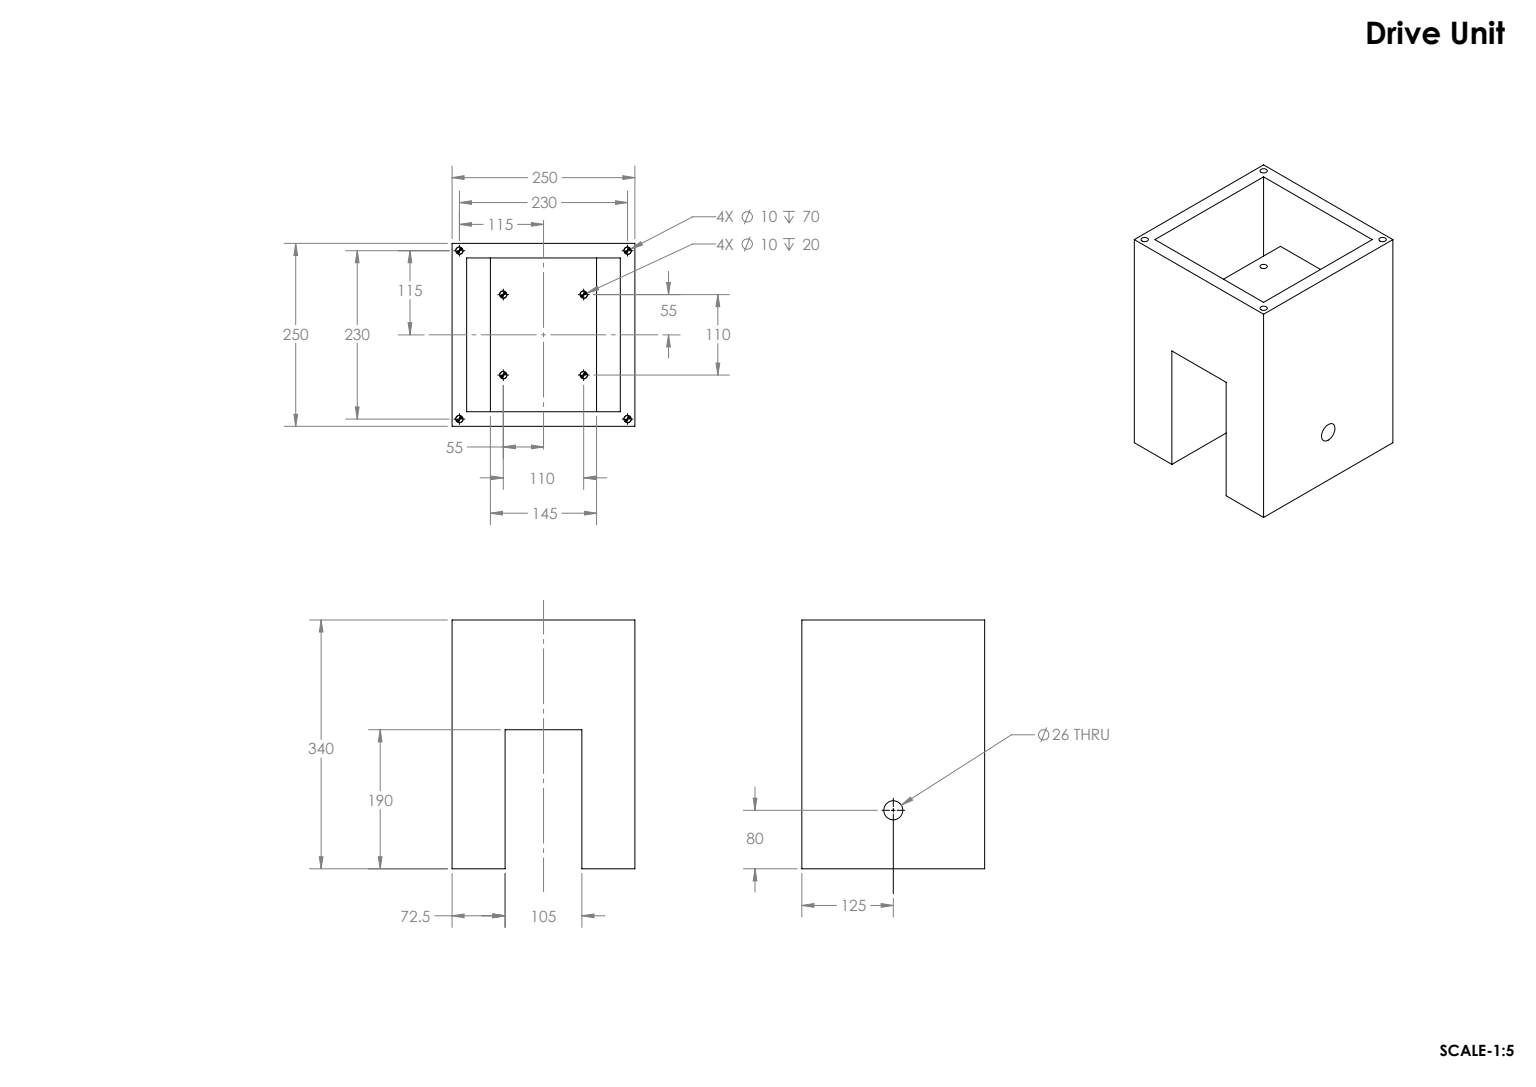
ISO-10303-21;
HEADER;
FILE_DESCRIPTION (('STEP AP214'),
    '1' );
FILE_NAME ('Drive Unit.step',
    '2026-10-28T15:55:38',
    ( '' ),
    ( '' ),
    'SwSTEP 2.0',
    'SolidWorks 2025',
    '' );
FILE_SCHEMA (( 'AUTOMOTIVE_DESIGN' ));
ENDSEC;

DATA;
#3=CARTESIAN_POINT ( 'NONE',  ( 125.0000000000000000, 52.50000000000000000, 190.0000000000000284 ) ) ;
#9=AXIS2_PLACEMENT_3D ( 'NONE', #2697, #3271, #106 ) ;
#13=ORIENTED_EDGE ( 'NONE', *, *, #6011, .T. ) ;
#17=CARTESIAN_POINT ( 'NONE',  ( 1.592040838891559490E-15, 125.0000000000000568, 92.99999999999992895 ) ) ;
#28=DIRECTION ( 'NONE',  ( -0.000000000000000000, -1.000000000000000000, 1.586032892321652236E-16 ) ) ;
#49=DIRECTION ( 'NONE',  ( -0.000000000000000000, -0.000000000000000000, 1.000000000000000000 ) ) ;
#55=ORIENTED_EDGE ( 'NONE', *, *, #309, .F. ) ;
#62=DIRECTION ( 'NONE',  ( -0.000000000000000000, -0.000000000000000000, 1.000000000000000000 ) ) ;
#63=FACE_OUTER_BOUND ( 'NONE', #5349, .T. ) ;
#67=VERTEX_POINT ( 'NONE', #6757 ) ;
#74=VECTOR ( 'NONE', #8127, 1000.000000000000000 ) ;
#78=LINE ( 'NONE', #2668, #2542 ) ;
#82=ORIENTED_EDGE ( 'NONE', *, *, #1098, .T. ) ;
#87=ADVANCED_FACE ( 'NONE', ( #1491 ), #7883, .F. ) ;
#93=DIRECTION ( 'NONE',  ( -0.000000000000000000, -1.460819769243626884E-16, -1.000000000000000000 ) ) ;
#94=SHAPE_REPRESENTATION_RELATIONSHIP ( 'NONE' , 'NONE' ,  #7203, #1812 ) ;
#98=VECTOR ( 'NONE', #4850, 1000.000000000000000 ) ;
#100=LINE ( 'NONE', #1995, #7998 ) ;
#102=DIRECTION ( 'NONE',  ( -0.000000000000000000, -0.000000000000000000, 1.000000000000000000 ) ) ;
#106=DIRECTION ( 'NONE',  ( 1.000000000000000000, 0.000000000000000000, 0.000000000000000000 ) ) ;
#109=CARTESIAN_POINT ( 'NONE',  ( -120.0000000000000000, 115.0000000000000000, 340.0000000000000000 ) ) ;
#112=VECTOR ( 'NONE', #2837, 1000.000000000000000 ) ;
#113=VECTOR ( 'NONE', #3248, 1000.000000000000000 ) ;
#120=CIRCLE ( 'NONE', #6870, 4.999999999999990230 ) ;
#123=FACE_OUTER_BOUND ( 'NONE', #4418, .T. ) ;
#124=ADVANCED_FACE ( 'NONE', ( #7222 ), #6594, .F. ) ;
#131=EDGE_CURVE ( 'NONE', #2948, #8274, #895, .T. ) ;
#136=CARTESIAN_POINT ( 'NONE',  ( -115.0000000000000142, 115.0000000000000000, 266.9956969048622568 ) ) ;
#137=ADVANCED_FACE ( 'NONE', ( #4082, #6676, #3444, #6029, #248 ), #2825, .F. ) ;
#145=DIRECTION ( 'NONE',  ( 1.000000000000000000, 0.000000000000000000, 0.000000000000000000 ) ) ;
#147=ORIENTED_EDGE ( 'NONE', *, *, #397, .F. ) ;
#149=DIRECTION ( 'NONE',  ( 0.000000000000000000, 0.000000000000000000, 1.000000000000000000 ) ) ;
#151=( NAMED_UNIT ( * ) PLANE_ANGLE_UNIT ( ) SI_UNIT ( $, .RADIAN. ) );
#152=EDGE_CURVE ( 'NONE', #6732, #6613, #6071, .T. ) ;
#157=ORIENTED_EDGE ( 'NONE', *, *, #4049, .T. ) ;
#162=DIRECTION ( 'NONE',  ( 0.000000000000000000, -1.224646799147353207E-16, 1.000000000000000000 ) ) ;
#164=DIRECTION ( 'NONE',  ( 0.000000000000000000, 1.224646799147353207E-16, -1.000000000000000000 ) ) ;
#168=CARTESIAN_POINT ( 'NONE',  ( -120.0000000000000000, 115.0000000000000000, 270.0000000000000000 ) ) ;
#171=CARTESIAN_POINT ( 'NONE',  ( 50.00000000000000711, 55.00000000000000000, 220.0000000000000284 ) ) ;
#174=CARTESIAN_POINT ( 'NONE',  ( -115.0000000000000000, 115.0000000000000000, 340.0000000000000000 ) ) ;
#184=LINE ( 'NONE', #4786, #3071 ) ;
#187=DIRECTION ( 'NONE',  ( -0.000000000000000000, -0.000000000000000000, 1.000000000000000000 ) ) ;
#193=ORIENTED_EDGE ( 'NONE', *, *, #2527, .T. ) ;
#199=DIRECTION ( 'NONE',  ( -0.000000000000000000, -1.632680918566406547E-16, -1.000000000000000000 ) ) ;
#205=( GEOMETRIC_REPRESENTATION_CONTEXT ( 3 ) GLOBAL_UNCERTAINTY_ASSIGNED_CONTEXT ( ( #320 ) ) GLOBAL_UNIT_ASSIGNED_CONTEXT ( ( #2718, #3942, #7322 ) ) REPRESENTATION_CONTEXT ( 'NONE', 'WORKASPACE' ) );
#214=DIRECTION ( 'NONE',  ( 1.000000000000000000, 0.000000000000000000, 0.000000000000000000 ) ) ;
#219=AXIS2_PLACEMENT_3D ( 'NONE', #1415, #5924, #6605 ) ;
#221=DIRECTION ( 'NONE',  ( -0.000000000000000000, -0.000000000000000000, 1.000000000000000000 ) ) ;
#223=ORIENTED_EDGE ( 'NONE', *, *, #4983, .T. ) ;
#224=CARTESIAN_POINT ( 'NONE',  ( 105.0000000000000000, 8.487013464091010249E-14, 20.00000000000001776 ) ) ;
#225=CARTESIAN_POINT ( 'NONE',  ( -125.0000000000000000, -125.0000000000000000, 340.0000000000000000 ) ) ;
#231=CONICAL_SURFACE ( 'NONE', #7932, 4.999999999999990230, 1.029744258676656754 ) ;
#233=PRODUCT_DEFINITION_CONTEXT ( 'detailed design', #2370, 'design' ) ;
#240=EDGE_CURVE ( 'NONE', #3849, #6134, #2101, .T. ) ;
#245=LINE ( 'NONE', #5564, #6769 ) ;
#247=CARTESIAN_POINT ( 'NONE',  ( 55.00000000000000000, 55.00000000000000000, 240.0000000000000284 ) ) ;
#248=FACE_OUTER_BOUND ( 'NONE', #5521, .T. ) ;
#255=CIRCLE ( 'NONE', #5116, 12.99999999999999822 ) ;
#256=DIRECTION ( 'NONE',  ( -1.000000000000000000, -1.321694076934710155E-16, 0.000000000000000000 ) ) ;
#260=VECTOR ( 'NONE', #1303, 1000.000000000000000 ) ;
#262=DIRECTION ( 'NONE',  ( -0.000000000000000000, -0.000000000000000000, 1.000000000000000000 ) ) ;
#264=EDGE_LOOP ( 'NONE', ( #6496, #2959, #7689, #1000 ) ) ;
#265=DIRECTION ( 'NONE',  ( 0.000000000000000000, 0.000000000000000000, -1.000000000000000000 ) ) ;
#266=LINE ( 'NONE', #3462, #5375 ) ;
#267=ORIENTED_EDGE ( 'NONE', *, *, #1486, .F. ) ;
#270=FACE_OUTER_BOUND ( 'NONE', #1601, .T. ) ;
#272=DIRECTION ( 'NONE',  ( 1.000000000000000000, 0.000000000000000000, 0.000000000000000000 ) ) ;
#276=CARTESIAN_POINT ( 'NONE',  ( -104.9999999999999432, -105.0000000000000853, 240.0000000000000284 ) ) ;
#279=CARTESIAN_POINT ( 'NONE',  ( 0.000000000000000000, 72.49999999999995737, 66.99999999999994316 ) ) ;
#287=CARTESIAN_POINT ( 'NONE',  ( 110.0000000000000142, -115.0000000000000000, 270.0000000000000000 ) ) ;
#289=CIRCLE ( 'NONE', #5015, 12.99999999999999822 ) ;
#292=ORIENTED_EDGE ( 'NONE', *, *, #3848, .F. ) ;
#297=PLANE ( 'NONE',  #642 ) ;
#303=CARTESIAN_POINT ( 'NONE',  ( 0.000000000000000000, 125.0000000000000568, 79.99999999999992895 ) ) ;
#309=EDGE_CURVE ( 'NONE', #7487, #6953, #643, .T. ) ;
#314=VERTEX_POINT ( 'NONE', #6672 ) ;
#320=UNCERTAINTY_MEASURE_WITH_UNIT (LENGTH_MEASURE( 1.000000000000000082E-05 ), #2718, 'distance_accuracy_value', 'NONE');
#323=VERTEX_POINT ( 'NONE', #4680 ) ;
#329=CARTESIAN_POINT ( 'NONE',  ( 120.0000000000000000, -115.0000000000000000, 270.0000000000000000 ) ) ;
#333=CARTESIAN_POINT ( 'NONE',  ( 125.0000000000000000, 52.50000000000000000, 190.0000000000000284 ) ) ;
#335=EDGE_CURVE ( 'NONE', #1946, #314, #6628, .T. ) ;
#336=ORIENTED_EDGE ( 'NONE', *, *, #3022, .F. ) ;
#344=CARTESIAN_POINT ( 'NONE',  ( 115.0000000000000000, 115.0000000000000000, 270.0000000000000000 ) ) ;
#345=DIRECTION ( 'NONE',  ( -0.000000000000000000, 1.000000000000000000, 1.224646799147353207E-16 ) ) ;
#346=EDGE_LOOP ( 'NONE', ( #3800, #3054, #6759, #1115 ) ) ;
#348=CARTESIAN_POINT ( 'NONE',  ( -115.0000000000000000, 115.0000000000000000, 340.0000000000000000 ) ) ;
#355=CARTESIAN_POINT ( 'NONE',  ( -110.0000000000000142, -115.0000000000000000, 270.0000000000000000 ) ) ;
#358=ORIENTED_EDGE ( 'NONE', *, *, #5305, .F. ) ;
#359=LINE ( 'NONE', #1094, #4691 ) ;
#360=ORIENTED_EDGE ( 'NONE', *, *, #2100, .T. ) ;
#366=DIRECTION ( 'NONE',  ( -0.000000000000000000, 1.000000000000000000, -0.000000000000000000 ) ) ;
#367=VECTOR ( 'NONE', #3652, 1000.000000000000000 ) ;
#368=ORIENTED_EDGE ( 'NONE', *, *, #2100, .F. ) ;
#373=CARTESIAN_POINT ( 'NONE',  ( 1.592040838891560279E-15, -125.0000000000000568, 92.99999999999997158 ) ) ;
#378=VERTEX_POINT ( 'NONE', #1356 ) ;
#385=EDGE_CURVE ( 'NONE', #378, #1211, #7861, .T. ) ;
#386=CARTESIAN_POINT ( 'NONE',  ( 105.0000000000000000, -105.0000000000000568, 240.0000000000000284 ) ) ;
#387=VECTOR ( 'NONE', #1755, 1000.000000000000000 ) ;
#397=EDGE_CURVE ( 'NONE', #2572, #1918, #4635, .T. ) ;
#416=VERTEX_POINT ( 'NONE', #5187 ) ;
#422=DIRECTION ( 'NONE',  ( -0.000000000000000000, -1.000000000000000000, -1.224646799147353207E-16 ) ) ;
#424=ORIENTED_EDGE ( 'NONE', *, *, #8219, .F. ) ;
#427=ORIENTED_EDGE ( 'NONE', *, *, #5038, .F. ) ;
#436=DIRECTION ( 'NONE',  ( -1.000000000000000000, -0.000000000000000000, -0.000000000000000000 ) ) ;
#439=DIRECTION ( 'NONE',  ( -0.000000000000000000, -0.000000000000000000, 1.000000000000000000 ) ) ;
#440=CARTESIAN_POINT ( 'NONE',  ( 1.592040838891560279E-15, -52.49999999999996447, 92.99999999999995737 ) ) ;
#443=EDGE_CURVE ( 'NONE', #5909, #448, #7758, .T. ) ;
#444=EDGE_CURVE ( 'NONE', #3837, #3210, #4518, .T. ) ;
#448=VERTEX_POINT ( 'NONE', #171 ) ;
#452=ORIENTED_EDGE ( 'NONE', *, *, #385, .T. ) ;
#454=ADVANCED_FACE ( 'NONE', ( #1334 ), #2234, .F. ) ;
#461=EDGE_CURVE ( 'NONE', #1211, #7416, #1823, .T. ) ;
#467=CARTESIAN_POINT ( 'NONE',  ( 0.000000000000000000, 72.49999999999995737, 79.99999999999994316 ) ) ;
#468=CYLINDRICAL_SURFACE ( 'NONE', #7813, 12.99999999999999822 ) ;
#469=VERTEX_POINT ( 'NONE', #7667 ) ;
#477=FACE_OUTER_BOUND ( 'NONE', #2938, .T. ) ;
#489=FACE_BOUND ( 'NONE', #5526, .T. ) ;
#503=DIRECTION ( 'NONE',  ( 1.000000000000000000, 1.321694076934710648E-16, 0.000000000000000000 ) ) ;
#508=ORIENTED_EDGE ( 'NONE', *, *, #4848, .F. ) ;
#509=VERTEX_POINT ( 'NONE', #329 ) ;
#510=EDGE_CURVE ( 'NONE', #4072, #3309, #2872, .T. ) ;
#513=DIRECTION ( 'NONE',  ( -0.000000000000000000, -0.000000000000000000, 1.000000000000000000 ) ) ;
#517=ORIENTED_EDGE ( 'NONE', *, *, #3189, .F. ) ;
#524=ORIENTED_EDGE ( 'NONE', *, *, #1693, .T. ) ;
#525=CIRCLE ( 'NONE', #6324, 4.999999999999990230 ) ;
#528=CARTESIAN_POINT ( 'NONE',  ( -55.00000000000000000, -55.00000000000000000, 220.0000000000000284 ) ) ;
#539=ORIENTED_EDGE ( 'NONE', *, *, #3641, .F. ) ;
#541=( GEOMETRIC_REPRESENTATION_CONTEXT ( 3 ) GLOBAL_UNCERTAINTY_ASSIGNED_CONTEXT ( ( #6320 ) ) GLOBAL_UNIT_ASSIGNED_CONTEXT ( ( #4638, #151, #7345 ) ) REPRESENTATION_CONTEXT ( 'NONE', 'WORKASPACE' ) );
#544=DIRECTION ( 'NONE',  ( -0.000000000000000000, -0.000000000000000000, 1.000000000000000000 ) ) ;
#549=VERTEX_POINT ( 'NONE', #6271 ) ;
#553=DIRECTION ( 'NONE',  ( -0.000000000000000000, -0.000000000000000000, 1.000000000000000000 ) ) ;
#556=CIRCLE ( 'NONE', #6891, 12.99999999999999822 ) ;
#564=CARTESIAN_POINT ( 'NONE',  ( -60.00000000000000000, 55.00000000000000000, 240.0000000000000284 ) ) ;
#568=DIRECTION ( 'NONE',  ( 1.000000000000000000, 0.000000000000000000, 0.000000000000000000 ) ) ;
#576=FACE_OUTER_BOUND ( 'NONE', #5063, .T. ) ;
#579=ADVANCED_FACE ( 'NONE', ( #2155 ), #2747, .F. ) ;
#580=ORIENTED_EDGE ( 'NONE', *, *, #3848, .T. ) ;
#591=ORIENTED_EDGE ( 'NONE', *, *, #4122, .F. ) ;
#603=LINE ( 'NONE', #4471, #650 ) ;
#605=DIRECTION ( 'NONE',  ( 1.000000000000000000, 0.000000000000000000, 0.000000000000000000 ) ) ;
#622=DIRECTION ( 'NONE',  ( -1.000000000000000000, 0.000000000000000000, -0.000000000000000000 ) ) ;
#623=ORIENTED_EDGE ( 'NONE', *, *, #2527, .F. ) ;
#624=VERTEX_POINT ( 'NONE', #5765 ) ;
#630=CARTESIAN_POINT ( 'NONE',  ( -105.0000000000000000, -72.49999999999994316, 20.00000000000002842 ) ) ;
#632=DIRECTION ( 'NONE',  ( 0.000000000000000000, -1.000000000000000000, 1.266875999117951024E-16 ) ) ;
#642=AXIS2_PLACEMENT_3D ( 'NONE', #2714, #6722, #256 ) ;
#643=LINE ( 'NONE', #4722, #6660 ) ;
#648=ORIENTED_EDGE ( 'NONE', *, *, #3135, .T. ) ;
#650=VECTOR ( 'NONE', #7306, 1000.000000000000000 ) ;
#651=ORIENTED_EDGE ( 'NONE', *, *, #7751, .F. ) ;
#657=PLANE ( 'NONE',  #5711 ) ;
#660=VECTOR ( 'NONE', #5010, 1000.000000000000000 ) ;
#679=VECTOR ( 'NONE', #7829, 1000.000000000000000 ) ;
#690=CARTESIAN_POINT ( 'NONE',  ( 0.000000000000000000, 72.49999999999995737, 79.99999999999994316 ) ) ;
#691=LINE ( 'NONE', #8174, #113 ) ;
#699=CARTESIAN_POINT ( 'NONE',  ( -55.00000000000000000, -55.00000000000000000, 220.0000000000000284 ) ) ;
#701=CARTESIAN_POINT ( 'NONE',  ( -60.00000000000000000, -55.00000000000000000, 240.0000000000000284 ) ) ;
#711=ORIENTED_EDGE ( 'NONE', *, *, #3187, .T. ) ;
#717=VERTEX_POINT ( 'NONE', #5434 ) ;
#726=CARTESIAN_POINT ( 'NONE',  ( 59.99999999999999289, 55.00000000000000000, 220.0000000000000284 ) ) ;
#728=DIRECTION ( 'NONE',  ( 0.000000000000000000, 0.000000000000000000, 1.000000000000000000 ) ) ;
#730=DIRECTION ( 'NONE',  ( -0.000000000000000000, 1.000000000000000000, 1.224646799147353207E-16 ) ) ;
#731=LINE ( 'NONE', #7181, #4203 ) ;
#736=CARTESIAN_POINT ( 'NONE',  ( 55.00000000000000000, 55.00000000000000000, 220.0000000000000284 ) ) ;
#746=FACE_OUTER_BOUND ( 'NONE', #7315, .T. ) ;
#747=EDGE_LOOP ( 'NONE', ( #539, #13, #8100 ) ) ;
#754=DIRECTION ( 'NONE',  ( 1.000000000000000000, 0.000000000000000000, 0.000000000000000000 ) ) ;
#762=DIRECTION ( 'NONE',  ( -1.000000000000000000, -0.000000000000000000, -0.000000000000000000 ) ) ;
#774=DIRECTION ( 'NONE',  ( 1.000000000000000000, 0.000000000000000000, 0.000000000000000000 ) ) ;
#782=DIRECTION ( 'NONE',  ( -0.000000000000000000, -0.000000000000000000, 1.000000000000000000 ) ) ;
#787=CIRCLE ( 'NONE', #5776, 4.999999999999997335 ) ;
#792=EDGE_CURVE ( 'NONE', #5384, #549, #5347, .T. ) ;
#798=FACE_BOUND ( 'NONE', #2089, .T. ) ;
#801=FACE_OUTER_BOUND ( 'NONE', #4380, .T. ) ;
#804=CARTESIAN_POINT ( 'NONE',  ( -115.0000000000000000, 115.0000000000000000, 340.0000000000000000 ) ) ;
#810=DIRECTION ( 'NONE',  ( 0.000000000000000000, -1.000000000000000000, -1.632680918566406547E-16 ) ) ;
#815=DIRECTION ( 'NONE',  ( -0.000000000000000000, -1.460819769243626884E-16, 1.000000000000000000 ) ) ;
#816=CIRCLE ( 'NONE', #7702, 4.999999999999990230 ) ;
#817=DIRECTION ( 'NONE',  ( 0.000000000000000000, 0.000000000000000000, -1.000000000000000000 ) ) ;
#821=DIRECTION ( 'NONE',  ( 1.000000000000000000, 0.000000000000000000, 0.000000000000000000 ) ) ;
#822=ORIENTED_EDGE ( 'NONE', *, *, #4122, .T. ) ;
#825=ORIENTED_EDGE ( 'NONE', *, *, #335, .F. ) ;
#839=LINE ( 'NONE', #6529, #4130 ) ;
#841=ORIENTED_EDGE ( 'NONE', *, *, #8140, .T. ) ;
#842=CIRCLE ( 'NONE', #983, 4.999999999999990230 ) ;
#851=CARTESIAN_POINT ( 'NONE',  ( 125.0000000000000000, -125.0000000000000000, 340.0000000000000000 ) ) ;
#852=DIRECTION ( 'NONE',  ( 1.000000000000000000, 0.000000000000000000, 0.000000000000000000 ) ) ;
#871=EDGE_CURVE ( 'NONE', #1109, #6237, #1148, .T. ) ;
#874=ADVANCED_FACE ( 'NONE', ( #1584 ), #2839, .F. ) ;
#876=DIRECTION ( 'NONE',  ( -0.000000000000000000, -1.460819769243626884E-16, 1.000000000000000000 ) ) ;
#879=CARTESIAN_POINT ( 'NONE',  ( 115.0000000000000000, 115.0000000000000000, 270.0000000000000000 ) ) ;
#884=ORIENTED_EDGE ( 'NONE', *, *, #4049, .F. ) ;
#889=CARTESIAN_POINT ( 'NONE',  ( 0.000000000000000000, -72.49999999999998579, 66.99999999999995737 ) ) ;
#890=PLANE ( 'NONE',  #4820 ) ;
#892=ADVANCED_FACE ( 'NONE', ( #5421 ), #4138, .F. ) ;
#895=LINE ( 'NONE', #5989, #5171 ) ;
#896=DIRECTION ( 'NONE',  ( 1.000000000000000000, 0.000000000000000000, 0.000000000000000000 ) ) ;
#903=FACE_OUTER_BOUND ( 'NONE', #8243, .T. ) ;
#907=VECTOR ( 'NONE', #3781, 1000.000000000000000 ) ;
#909=ORIENTED_EDGE ( 'NONE', *, *, #2279, .F. ) ;
#915=CARTESIAN_POINT ( 'NONE',  ( -105.0000000000000000, 8.487013464091010249E-14, 20.00000000000001776 ) ) ;
#922=EDGE_CURVE ( 'NONE', #6580, #3406, #3545, .T. ) ;
#923=VECTOR ( 'NONE', #513, 1000.000000000000000 ) ;
#942=DIRECTION ( 'NONE',  ( 0.000000000000000000, 0.000000000000000000, -1.000000000000000000 ) ) ;
#944=VECTOR ( 'NONE', #2401, 1000.000000000000000 ) ;
#952=VERTEX_POINT ( 'NONE', #3626 ) ;
#954=DIRECTION ( 'NONE',  ( 1.000000000000000000, 0.000000000000000000, 0.000000000000000000 ) ) ;
#962=EDGE_LOOP ( 'NONE', ( #5950, #591, #6803, #1518 ) ) ;
#963=ORIENTED_EDGE ( 'NONE', *, *, #1804, .T. ) ;
#972=ORIENTED_EDGE ( 'NONE', *, *, #2430, .F. ) ;
#977=DIRECTION ( 'NONE',  ( -0.000000000000000000, -0.000000000000000000, 1.000000000000000000 ) ) ;
#982=ADVANCED_FACE ( 'NONE', ( #4567 ), #7087, .F. ) ;
#983=AXIS2_PLACEMENT_3D ( 'NONE', #7682, #6478, #5268 ) ;
#1000=ORIENTED_EDGE ( 'NONE', *, *, #4569, .F. ) ;
#1001=DIRECTION ( 'NONE',  ( 1.000000000000000000, 0.000000000000000000, 0.000000000000000000 ) ) ;
#1008=VERTEX_POINT ( 'NONE', #7708 ) ;
#1017=DIRECTION ( 'NONE',  ( 0.000000000000000000, -1.224646799147353207E-16, 1.000000000000000000 ) ) ;
#1029=PLANE ( 'NONE',  #4537 ) ;
#1032=ORIENTED_EDGE ( 'NONE', *, *, #7372, .F. ) ;
#1033=AXIS2_PLACEMENT_3D ( 'NONE', #4475, #7026, #568 ) ;
#1034=ORIENTED_EDGE ( 'NONE', *, *, #3154, .F. ) ;
#1037=CARTESIAN_POINT ( 'NONE',  ( -115.0000000000000000, -115.0000000000000000, 340.0000000000000000 ) ) ;
#1038=ORIENTED_EDGE ( 'NONE', *, *, #5870, .T. ) ;
#1042=DIRECTION ( 'NONE',  ( 1.000000000000000000, 0.000000000000000000, 0.000000000000000000 ) ) ;
#1044=ORIENTED_EDGE ( 'NONE', *, *, #5451, .F. ) ;
#1050=CARTESIAN_POINT ( 'NONE',  ( -50.00000000000000000, -55.00000000000000000, 240.0000000000000284 ) ) ;
#1061=CARTESIAN_POINT ( 'NONE',  ( -105.0000000000000000, 8.487013464091010249E-14, 20.00000000000001776 ) ) ;
#1062=ORIENTED_EDGE ( 'NONE', *, *, #4848, .T. ) ;
#1067=EDGE_LOOP ( 'NONE', ( #3144, #1132, #360, #4244, #5256, #6664, #7467, #3226 ) ) ;
#1070=DIRECTION ( 'NONE',  ( 0.000000000000000000, 1.000000000000000000, -1.460819769243626884E-16 ) ) ;
#1082=AXIS2_PLACEMENT_3D ( 'NONE', #3202, #6495, #7747 ) ;
#1088=CARTESIAN_POINT ( 'NONE',  ( 0.000000000000000000, 125.0000000000000568, 79.99999999999992895 ) ) ;
#1093=VERTEX_POINT ( 'NONE', #4424 ) ;
#1094=CARTESIAN_POINT ( 'NONE',  ( 0.000000000000000000, 105.0000000000000568, 19.99999999999998934 ) ) ;
#1095=DIRECTION ( 'NONE',  ( 1.000000000000000000, 0.000000000000000000, 0.000000000000000000 ) ) ;
#1098=EDGE_CURVE ( 'NONE', #448, #3289, #5832, .T. ) ;
#1103=LINE ( 'NONE', #3662, #3498 ) ;
#1107=VECTOR ( 'NONE', #2087, 1000.000000000000000 ) ;
#1109=VERTEX_POINT ( 'NONE', #1317 ) ;
#1110=CARTESIAN_POINT ( 'NONE',  ( 110.0000000000000142, 115.0000000000000000, 270.0000000000000000 ) ) ;
#1112=VERTEX_POINT ( 'NONE', #1965 ) ;
#1115=ORIENTED_EDGE ( 'NONE', *, *, #3920, .T. ) ;
#1120=ORIENTED_EDGE ( 'NONE', *, *, #6894, .T. ) ;
#1122=DIRECTION ( 'NONE',  ( 0.000000000000000000, 0.000000000000000000, -1.000000000000000000 ) ) ;
#1123=VECTOR ( 'NONE', #1801, 1000.000000000000000 ) ;
#1132=ORIENTED_EDGE ( 'NONE', *, *, #5688, .T. ) ;
#1141=DIRECTION ( 'NONE',  ( 1.321694076934710648E-16, -1.000000000000000000, 0.000000000000000000 ) ) ;
#1148=CIRCLE ( 'NONE', #5858, 4.999999999999990230 ) ;
#1155=ORIENTED_EDGE ( 'NONE', *, *, #7137, .F. ) ;
#1166=LINE ( 'NONE', #2919, #1123 ) ;
#1168=DIRECTION ( 'NONE',  ( 1.000000000000000000, 0.000000000000000000, 0.000000000000000000 ) ) ;
#1195=ORIENTED_EDGE ( 'NONE', *, *, #7394, .T. ) ;
#1206=DIRECTION ( 'NONE',  ( -0.000000000000000000, -0.000000000000000000, 1.000000000000000000 ) ) ;
#1211=VERTEX_POINT ( 'NONE', #1443 ) ;
#1212=CARTESIAN_POINT ( 'NONE',  ( 1.592040838891560279E-15, 52.49999999999997868, 92.99999999999994316 ) ) ;
#1213=CIRCLE ( 'NONE', #4702, 12.99999999999999822 ) ;
#1218=CARTESIAN_POINT ( 'NONE',  ( 115.0000000000000000, -115.0000000000000000, 340.0000000000000000 ) ) ;
#1219=DIRECTION ( 'NONE',  ( 1.000000000000000000, 0.000000000000000000, 0.000000000000000000 ) ) ;
#1228=ORIENTED_EDGE ( 'NONE', *, *, #4164, .F. ) ;
#1231=PLANE ( 'NONE',  #1375 ) ;
#1232=ORIENTED_EDGE ( 'NONE', *, *, #6853, .T. ) ;
#1238=EDGE_LOOP ( 'NONE', ( #1678, #6258, #1261 ) ) ;
#1239=ORIENTED_EDGE ( 'NONE', *, *, #6373, .T. ) ;
#1243=EDGE_LOOP ( 'NONE', ( #8310, #7332 ) ) ;
#1244=AXIS2_PLACEMENT_3D ( 'NONE', #7131, #1351, #3234 ) ;
#1247=DIRECTION ( 'NONE',  ( 0.000000000000000000, 0.000000000000000000, 1.000000000000000000 ) ) ;
#1249=DIRECTION ( 'NONE',  ( 0.000000000000000000, -1.224646799147353207E-16, 1.000000000000000000 ) ) ;
#1250=ORIENTED_EDGE ( 'NONE', *, *, #444, .F. ) ;
#1251=DIRECTION ( 'NONE',  ( 0.000000000000000000, -1.000000000000000000, 1.586032892321652236E-16 ) ) ;
#1261=ORIENTED_EDGE ( 'NONE', *, *, #871, .T. ) ;
#1266=CARTESIAN_POINT ( 'NONE',  ( 110.0000000000000142, 115.0000000000000000, 270.0000000000000000 ) ) ;
#1279=DIRECTION ( 'NONE',  ( -1.000000000000000000, 0.000000000000000000, 0.000000000000000000 ) ) ;
#1283=EDGE_CURVE ( 'NONE', #5670, #323, #4893, .T. ) ;
#1289=DIRECTION ( 'NONE',  ( -0.000000000000000000, 1.266875999117951024E-16, 1.000000000000000000 ) ) ;
#1297=ORIENTED_EDGE ( 'NONE', *, *, #4699, .T. ) ;
#1299=AXIS2_PLACEMENT_3D ( 'NONE', #5884, #1507, #5927 ) ;
#1301=DIRECTION ( 'NONE',  ( 1.000000000000000000, 0.000000000000000000, 0.000000000000000000 ) ) ;
#1303=DIRECTION ( 'NONE',  ( -0.000000000000000000, -0.000000000000000000, 1.000000000000000000 ) ) ;
#1312=CARTESIAN_POINT ( 'NONE',  ( 0.000000000000000000, 125.0000000000000568, 79.99999999999992895 ) ) ;
#1317=CARTESIAN_POINT ( 'NONE',  ( 120.0000000000000000, 115.0000000000000000, 270.0000000000000000 ) ) ;
#1318=AXIS2_PLACEMENT_3D ( 'NONE', #2518, #49, #5807 ) ;
#1323=CARTESIAN_POINT ( 'NONE',  ( -55.00000000000000000, -55.00000000000000000, 240.0000000000000284 ) ) ;
#1324=CARTESIAN_POINT ( 'NONE',  ( 0.000000000000000000, 125.0000000000000568, 79.99999999999992895 ) ) ;
#1325=ORIENTED_EDGE ( 'NONE', *, *, #5972, .F. ) ;
#1326=FACE_OUTER_BOUND ( 'NONE', #4672, .T. ) ;
#1334=FACE_OUTER_BOUND ( 'NONE', #3551, .T. ) ;
#1337=CYLINDRICAL_SURFACE ( 'NONE', #2260, 12.99999999999999822 ) ;
#1342=ORIENTED_EDGE ( 'NONE', *, *, #2323, .F. ) ;
#1343=EDGE_CURVE ( 'NONE', #469, #717, #245, .T. ) ;
#1350=LINE ( 'NONE', #1266, #7264 ) ;
#1351=DIRECTION ( 'NONE',  ( -0.000000000000000000, -0.000000000000000000, 1.000000000000000000 ) ) ;
#1353=ORIENTED_EDGE ( 'NONE', *, *, #6378, .F. ) ;
#1355=ORIENTED_EDGE ( 'NONE', *, *, #1343, .T. ) ;
#1356=CARTESIAN_POINT ( 'NONE',  ( 54.99999999999999289, -55.00000000000000000, 216.9956969048622284 ) ) ;
#1357=EDGE_CURVE ( 'NONE', #3406, #6580, #842, .T. ) ;
#1369=CARTESIAN_POINT ( 'NONE',  ( 0.000000000000000000, 52.49999999999997868, 79.99999999999994316 ) ) ;
#1375=AXIS2_PLACEMENT_3D ( 'NONE', #6364, #3156, #632 ) ;
#1379=CARTESIAN_POINT ( 'NONE',  ( -59.99999999999999289, 55.00000000000000000, 220.0000000000000284 ) ) ;
#1383=ORIENTED_EDGE ( 'NONE', *, *, #1921, .F. ) ;
#1391=DIRECTION ( 'NONE',  ( -1.000000000000000000, -0.000000000000000000, 0.000000000000000000 ) ) ;
#1395=DIRECTION ( 'NONE',  ( -0.000000000000000000, -1.000000000000000000, -1.224646799147353207E-16 ) ) ;
#1415=CARTESIAN_POINT ( 'NONE',  ( 55.00000000000000000, -55.00000000000000000, 220.0000000000000284 ) ) ;
#1416=DIRECTION ( 'NONE',  ( 1.000000000000000000, 0.000000000000000000, 0.000000000000000000 ) ) ;
#1428=CYLINDRICAL_SURFACE ( 'NONE', #5906, 4.999999999999997335 ) ;
#1429=CARTESIAN_POINT ( 'NONE',  ( -55.00000000000000000, 55.00000000000000000, 240.0000000000000284 ) ) ;
#1443=CARTESIAN_POINT ( 'NONE',  ( 59.99999999999999289, -55.00000000000000000, 220.0000000000000284 ) ) ;
#1445=DIRECTION ( 'NONE',  ( -0.000000000000000000, -0.000000000000000000, 1.000000000000000000 ) ) ;
#1451=LINE ( 'NONE', #2709, #7830 ) ;
#1458=CARTESIAN_POINT ( 'NONE',  ( 125.0000000000000000, 52.49999999999997158, 0.000000000000000000 ) ) ;
#1459=DIRECTION ( 'NONE',  ( -0.000000000000000000, -0.000000000000000000, 1.000000000000000000 ) ) ;
#1469=CARTESIAN_POINT ( 'NONE',  ( -55.00000000000000000, -55.00000000000000000, 220.0000000000000284 ) ) ;
#1475=AXIS2_PLACEMENT_3D ( 'NONE', #1369, #3932, #5873 ) ;
#1480=AXIS2_PLACEMENT_3D ( 'NONE', #386, #2871, #1541 ) ;
#1486=EDGE_CURVE ( 'NONE', #3309, #4072, #289, .T. ) ;
#1489=CARTESIAN_POINT ( 'NONE',  ( -125.0000000000000000, -52.50000000000000000, 190.0000000000000284 ) ) ;
#1491=FACE_OUTER_BOUND ( 'NONE', #747, .T. ) ;
#1496=EDGE_LOOP ( 'NONE', ( #3327, #3854, #5221 ) ) ;
#1507=DIRECTION ( 'NONE',  ( 0.000000000000000000, 0.000000000000000000, 1.000000000000000000 ) ) ;
#1512=CIRCLE ( 'NONE', #6214, 4.999999999999990230 ) ;
#1518=ORIENTED_EDGE ( 'NONE', *, *, #5972, .T. ) ;
#1520=ORIENTED_EDGE ( 'NONE', *, *, #3187, .F. ) ;
#1534=VERTEX_POINT ( 'NONE', #2242 ) ;
#1536=AXIS2_PLACEMENT_3D ( 'NONE', #4125, #942, #3490 ) ;
#1539=DIRECTION ( 'NONE',  ( 1.000000000000000000, 0.000000000000000000, 0.000000000000000000 ) ) ;
#1541=DIRECTION ( 'NONE',  ( 0.000000000000000000, 0.000000000000000000, -1.000000000000000000 ) ) ;
#1544=LINE ( 'NONE', #6081, #387 ) ;
#1547=LINE ( 'NONE', #2193, #3061 ) ;
#1551=FACE_OUTER_BOUND ( 'NONE', #7596, .T. ) ;
#1553=ORIENTED_EDGE ( 'NONE', *, *, #1693, .F. ) ;
#1556=EDGE_CURVE ( 'NONE', #1093, #3982, #1166, .T. ) ;
#1562=VERTEX_POINT ( 'NONE', #8172 ) ;
#1571=DIRECTION ( 'NONE',  ( 0.000000000000000000, -1.224646799147353207E-16, 1.000000000000000000 ) ) ;
#1575=DIRECTION ( 'NONE',  ( -0.000000000000000000, 1.266875999117951024E-16, 1.000000000000000000 ) ) ;
#1584=FACE_OUTER_BOUND ( 'NONE', #7774, .T. ) ;
#1588=ORIENTED_EDGE ( 'NONE', *, *, #3237, .T. ) ;
#1591=AXIS2_PLACEMENT_3D ( 'NONE', #3931, #5710, #6978 ) ;
#1596=CARTESIAN_POINT ( 'NONE',  ( -55.00000000000000000, -55.00000000000000000, 220.0000000000000284 ) ) ;
#1597=AXIS2_PLACEMENT_3D ( 'NONE', #4723, #1445, #2133 ) ;
#1601=EDGE_LOOP ( 'NONE', ( #2907, #8094, #822 ) ) ;
#1604=AXIS2_PLACEMENT_3D ( 'NONE', #4532, #7083, #1301 ) ;
#1622=AXIS2_PLACEMENT_3D ( 'NONE', #2587, #6337, #5791 ) ;
#1628=DIRECTION ( 'NONE',  ( 0.000000000000000000, 0.000000000000000000, -1.000000000000000000 ) ) ;
#1629=FACE_OUTER_BOUND ( 'NONE', #264, .T. ) ;
#1630=ORIENTED_EDGE ( 'NONE', *, *, #7051, .T. ) ;
#1637=ORIENTED_EDGE ( 'NONE', *, *, #444, .T. ) ;
#1643=EDGE_CURVE ( 'NONE', #6249, #5775, #7359, .T. ) ;
#1647=EDGE_CURVE ( 'NONE', #4789, #3289, #5301, .T. ) ;
#1648=ORIENTED_EDGE ( 'NONE', *, *, #5870, .F. ) ;
#1649=DIRECTION ( 'NONE',  ( 0.8571673007021134438, 0.000000000000000000, 0.5150380749100522682 ) ) ;
#1658=FACE_OUTER_BOUND ( 'NONE', #1067, .T. ) ;
#1665=VERTEX_POINT ( 'NONE', #7350 ) ;
#1671=EDGE_LOOP ( 'NONE', ( #3004, #2889, #8068, #4799 ) ) ;
#1672=CYLINDRICAL_SURFACE ( 'NONE', #4564, 12.99999999999999822 ) ;
#1676=DIRECTION ( 'NONE',  ( 1.000000000000000000, 0.000000000000000000, 0.000000000000000000 ) ) ;
#1678=ORIENTED_EDGE ( 'NONE', *, *, #6853, .F. ) ;
#1690=CARTESIAN_POINT ( 'NONE',  ( -115.0000000000000000, -115.0000000000000000, 270.0000000000000000 ) ) ;
#1693=EDGE_CURVE ( 'NONE', #5775, #2457, #5565, .T. ) ;
#1709=AXIS2_PLACEMENT_3D ( 'NONE', #4046, #7188, #5252 ) ;
#1710=ORIENTED_EDGE ( 'NONE', *, *, #6741, .T. ) ;
#1716=CARTESIAN_POINT ( 'NONE',  ( -115.0000000000000000, 115.0000000000000000, 270.0000000000000000 ) ) ;
#1722=ORIENTED_EDGE ( 'NONE', *, *, #7897, .T. ) ;
#1723=LINE ( 'NONE', #4756, #3086 ) ;
#1726=CARTESIAN_POINT ( 'NONE',  ( 125.0000000000000000, 125.0000000000000568, -9.184850993605156622E-15 ) ) ;
#1736=VECTOR ( 'NONE', #7864, 1000.000000000000000 ) ;
#1737=ORIENTED_EDGE ( 'NONE', *, *, #443, .F. ) ;
#1753=LINE ( 'NONE', #2434, #2301 ) ;
#1755=DIRECTION ( 'NONE',  ( -1.000000000000000000, 0.000000000000000000, 0.000000000000000000 ) ) ;
#1757=ADVANCED_FACE ( 'NONE', ( #3722 ), #3166, .F. ) ;
#1759=EDGE_CURVE ( 'NONE', #3837, #1946, #3323, .T. ) ;
#1775=CARTESIAN_POINT ( 'NONE',  ( 0.000000000000000000, -125.0000000000000568, 79.99999999999997158 ) ) ;
#1782=ORIENTED_EDGE ( 'NONE', *, *, #6074, .T. ) ;
#1786=AXIS2_PLACEMENT_3D ( 'NONE', #8007, #8046, #272 ) ;
#1796=CARTESIAN_POINT ( 'NONE',  ( 105.0000000000000000, -105.0000000000000568, 240.0000000000000284 ) ) ;
#1801=DIRECTION ( 'NONE',  ( 1.000000000000000000, 0.000000000000000000, 0.000000000000000000 ) ) ;
#1804=EDGE_CURVE ( 'NONE', #378, #7416, #731, .T. ) ;
#1806=EDGE_CURVE ( 'NONE', #4162, #3924, #4896, .T. ) ;
#1809=VECTOR ( 'NONE', #3841, 1000.000000000000000 ) ;
#1810=ORIENTED_EDGE ( 'NONE', *, *, #5085, .T. ) ;
#1812=ADVANCED_BREP_SHAPE_REPRESENTATION ( '', ( #6502, #1299 ), #205 ) ;
#1816=ORIENTED_EDGE ( 'NONE', *, *, #1283, .T. ) ;
#1819=CARTESIAN_POINT ( 'NONE',  ( 120.0000000000000000, -115.0000000000000000, 340.0000000000000000 ) ) ;
#1823=CIRCLE ( 'NONE', #3960, 4.999999999999990230 ) ;
#1837=ORIENTED_EDGE ( 'NONE', *, *, #3482, .T. ) ;
#1839=FACE_OUTER_BOUND ( 'NONE', #7122, .T. ) ;
#1840=DIRECTION ( 'NONE',  ( -0.000000000000000000, -1.000000000000000000, 1.586032892321652236E-16 ) ) ;
#1847=DIRECTION ( 'NONE',  ( -0.000000000000000000, -1.000000000000000000, 1.586032892321652236E-16 ) ) ;
#1857=DIRECTION ( 'NONE',  ( -0.8571673007021116675, 1.049727191138617833E-16, 0.5150380749100552658 ) ) ;
#1862=ORIENTED_EDGE ( 'NONE', *, *, #6074, .F. ) ;
#1872=CARTESIAN_POINT ( 'NONE',  ( 120.0000000000000000, -115.0000000000000000, 340.0000000000000000 ) ) ;
#1875=LINE ( 'NONE', #5150, #6737 ) ;
#1877=AXIS2_PLACEMENT_3D ( 'NONE', #1596, #5896, #7892 ) ;
#1878=VERTEX_POINT ( 'NONE', #6800 ) ;
#1893=CIRCLE ( 'NONE', #2163, 4.999999999999990230 ) ;
#1904=VERTEX_POINT ( 'NONE', #7572 ) ;
#1911=ORIENTED_EDGE ( 'NONE', *, *, #7216, .T. ) ;
#1918=VERTEX_POINT ( 'NONE', #7219 ) ;
#1921=EDGE_CURVE ( 'NONE', #67, #5909, #2099, .T. ) ;
#1922=ADVANCED_FACE ( 'NONE', ( #2703, #5284 ), #890, .F. ) ;
#1929=DIRECTION ( 'NONE',  ( -0.000000000000000000, 0.000000000000000000, 1.000000000000000000 ) ) ;
#1935=VERTEX_POINT ( 'NONE', #5949 ) ;
#1946=VERTEX_POINT ( 'NONE', #4719 ) ;
#1950=CARTESIAN_POINT ( 'NONE',  ( -50.00000000000000711, -55.00000000000000000, 220.0000000000000284 ) ) ;
#1951=EDGE_LOOP ( 'NONE', ( #3758, #5816, #825, #2312 ) ) ;
#1953=CARTESIAN_POINT ( 'NONE',  ( 1.592040838891559490E-15, 125.0000000000000568, 92.99999999999992895 ) ) ;
#1954=CARTESIAN_POINT ( 'NONE',  ( -104.9999999999999432, -105.0000000000000853, 240.0000000000000284 ) ) ;
#1960=CARTESIAN_POINT ( 'NONE',  ( 59.99999999999999289, -55.00000000000000000, 220.0000000000000284 ) ) ;
#1961=CYLINDRICAL_SURFACE ( 'NONE', #4815, 4.999999999999990230 ) ;
#1964=DIRECTION ( 'NONE',  ( 1.000000000000000000, 0.000000000000000000, 0.000000000000000000 ) ) ;
#1965=CARTESIAN_POINT ( 'NONE',  ( -120.0000000000000000, 115.0000000000000000, 270.0000000000000000 ) ) ;
#1972=CARTESIAN_POINT ( 'NONE',  ( 0.000000000000000000, -72.49999999999994316, -212.5000000000000568 ) ) ;
#1974=ORIENTED_EDGE ( 'NONE', *, *, #2868, .T. ) ;
#1995=CARTESIAN_POINT ( 'NONE',  ( 125.0000000000000000, -52.50000000000000000, 190.0000000000000284 ) ) ;
#1997=ORIENTED_EDGE ( 'NONE', *, *, #2026, .T. ) ;
#2004=CARTESIAN_POINT ( 'NONE',  ( 55.00000000000000000, 55.00000000000000000, 220.0000000000000284 ) ) ;
#2006=ORIENTED_EDGE ( 'NONE', *, *, #8312, .F. ) ;
#2012=CARTESIAN_POINT ( 'NONE',  ( 105.0000000000000000, 72.49999999999994316, 240.0000000000000284 ) ) ;
#2014=CIRCLE ( 'NONE', #6979, 12.99999999999999822 ) ;
#2020=DIRECTION ( 'NONE',  ( -0.8571673007021134438, 1.049727191138620051E-16, 0.5150380749100522682 ) ) ;
#2026=EDGE_CURVE ( 'NONE', #6580, #5343, #5986, .T. ) ;
#2031=AXIS2_PLACEMENT_3D ( 'NONE', #2189, #4740, #7321 ) ;
#2032=EDGE_CURVE ( 'NONE', #6276, #1109, #7478, .T. ) ;
#2035=CARTESIAN_POINT ( 'NONE',  ( -105.0000000000000000, 72.49999999999994316, 240.0000000000000284 ) ) ;
#2049=CARTESIAN_POINT ( 'NONE',  ( 55.00000000000000000, -55.00000000000000000, 240.0000000000000284 ) ) ;
#2051=EDGE_LOOP ( 'NONE', ( #4977, #6871 ) ) ;
#2057=ORIENTED_EDGE ( 'NONE', *, *, #4536, .F. ) ;
#2067=CARTESIAN_POINT ( 'NONE',  ( -120.0000000000000000, -115.0000000000000000, 340.0000000000000000 ) ) ;
#2072=CARTESIAN_POINT ( 'NONE',  ( -125.0000000000000000, 52.50000000000000000, 190.0000000000000284 ) ) ;
#2074=CARTESIAN_POINT ( 'NONE',  ( 125.0000000000000000, -52.49999999999997158, 0.000000000000000000 ) ) ;
#2081=EDGE_LOOP ( 'NONE', ( #147, #6748, #1034, #3870, #55, #6533, #2869, #3571 ) ) ;
#2087=DIRECTION ( 'NONE',  ( 0.8571673007021134438, 0.000000000000000000, 0.5150380749100522682 ) ) ;
#2088=EDGE_CURVE ( 'NONE', #2457, #5057, #5401, .T. ) ;
#2089=EDGE_LOOP ( 'NONE', ( #2586, #7609 ) ) ;
#2099=LINE ( 'NONE', #726, #1736 ) ;
#2100=EDGE_CURVE ( 'NONE', #469, #8240, #4120, .T. ) ;
#2101=CIRCLE ( 'NONE', #4632, 12.99999999999999822 ) ;
#2105=EDGE_CURVE ( 'NONE', #5395, #2109, #556, .T. ) ;
#2106=CARTESIAN_POINT ( 'NONE',  ( -55.00000000000000000, 55.00000000000000000, 240.0000000000000284 ) ) ;
#2109=VERTEX_POINT ( 'NONE', #2259 ) ;
#2113=CARTESIAN_POINT ( 'NONE',  ( -104.9999999999999432, -105.0000000000000853, 240.0000000000000284 ) ) ;
#2124=AXIS2_PLACEMENT_3D ( 'NONE', #6427, #3220, #2606 ) ;
#2127=CIRCLE ( 'NONE', #6821, 4.999999999999997335 ) ;
#2131=VECTOR ( 'NONE', #8255, 1000.000000000000000 ) ;
#2133=DIRECTION ( 'NONE',  ( 1.000000000000000000, 0.000000000000000000, 0.000000000000000000 ) ) ;
#2144=VECTOR ( 'NONE', #28, 1000.000000000000000 ) ;
#2155=FACE_OUTER_BOUND ( 'NONE', #1496, .T. ) ;
#2156=ORIENTED_EDGE ( 'NONE', *, *, #4836, .T. ) ;
#2158=DIRECTION ( 'NONE',  ( -0.000000000000000000, -0.000000000000000000, 1.000000000000000000 ) ) ;
#2160=VECTOR ( 'NONE', #1857, 1000.000000000000000 ) ;
#2163=AXIS2_PLACEMENT_3D ( 'NONE', #528, #8221, #1168 ) ;
#2164=EDGE_CURVE ( 'NONE', #6732, #509, #7739, .T. ) ;
#2167=ORIENTED_EDGE ( 'NONE', *, *, #4580, .T. ) ;
#2171=ADVANCED_FACE ( 'NONE', ( #4410 ), #1231, .T. ) ;
#2172=EDGE_CURVE ( 'NONE', #1878, #7656, #1103, .T. ) ;
#2173=CARTESIAN_POINT ( 'NONE',  ( 60.00000000000000000, 55.00000000000000000, 240.0000000000000284 ) ) ;
#2175=AXIS2_PLACEMENT_3D ( 'NONE', #1726, #1575, #3608 ) ;
#2176=DIRECTION ( 'NONE',  ( 0.000000000000000000, 0.000000000000000000, -1.000000000000000000 ) ) ;
#2177=CARTESIAN_POINT ( 'NONE',  ( -115.0000000000000000, 115.0000000000000000, 270.0000000000000000 ) ) ;
#2182=ORIENTED_EDGE ( 'NONE', *, *, #3572, .F. ) ;
#2189=CARTESIAN_POINT ( 'NONE',  ( -115.0000000000000000, 115.0000000000000000, 270.0000000000000000 ) ) ;
#2190=VECTOR ( 'NONE', #366, 1000.000000000000000 ) ;
#2193=CARTESIAN_POINT ( 'NONE',  ( 105.0000000000000000, -105.0000000000000568, 240.0000000000000284 ) ) ;
#2199=EDGE_LOOP ( 'NONE', ( #7443, #8010, #5457 ) ) ;
#2203=DIRECTION ( 'NONE',  ( 0.000000000000000000, -1.000000000000000000, -1.460819769243626884E-16 ) ) ;
#2206=EDGE_LOOP ( 'NONE', ( #2331, #1250, #6833, #157 ) ) ;
#2230=CLOSED_SHELL ( 'NONE', ( #7292, #3818, #3695, #7103, #892, #4170, #7703, #2485, #7938, #579, #5920, #3689, #2276, #4404, #6905, #7013, #3012, #1757, #8269, #874, #137, #7115, #5151, #2721, #6602, #124, #3198, #4584, #3574, #8030, #1922, #2630, #6400, #4513, #2249, #7480, #6634, #7438, #4322, #3235, #7023, #2366, #4996, #982, #4732, #3586, #2579, #6350, #4357, #454, #5774, #3175, #5137, #87, #5192, #7718, #2171, #2926, #7211 ) ) ;
#2234=CONICAL_SURFACE ( 'NONE', #7068, 4.999999999999990230, 1.029744258676656754 ) ;
#2242=CARTESIAN_POINT ( 'NONE',  ( 110.0000000000000142, -115.0000000000000000, 340.0000000000000000 ) ) ;
#2244=ORIENTED_EDGE ( 'NONE', *, *, #7704, .F. ) ;
#2245=DIRECTION ( 'NONE',  ( 1.000000000000000000, 0.000000000000000000, 0.000000000000000000 ) ) ;
#2248=FACE_OUTER_BOUND ( 'NONE', #5783, .T. ) ;
#2249=ADVANCED_FACE ( 'NONE', ( #7931 ), #5823, .T. ) ;
#2251=CARTESIAN_POINT ( 'NONE',  ( 115.0000000000000000, -115.0000000000000000, 270.0000000000000000 ) ) ;
#2254=DIRECTION ( 'NONE',  ( -1.000000000000000000, 0.000000000000000000, 0.000000000000000000 ) ) ;
#2259=CARTESIAN_POINT ( 'NONE',  ( 1.592040838891560279E-15, 105.0000000000000426, 92.99999999999992895 ) ) ;
#2260=AXIS2_PLACEMENT_3D ( 'NONE', #3141, #1847, #7677 ) ;
#2268=EDGE_CURVE ( 'NONE', #1008, #7487, #3989, .T. ) ;
#2276=ADVANCED_FACE ( 'NONE', ( #2658 ), #2766, .F. ) ;
#2279=EDGE_CURVE ( 'NONE', #8276, #5343, #7442, .T. ) ;
#2280=DIRECTION ( 'NONE',  ( -0.000000000000000000, -0.000000000000000000, 1.000000000000000000 ) ) ;
#2281=ORIENTED_EDGE ( 'NONE', *, *, #4563, .F. ) ;
#2284=CARTESIAN_POINT ( 'NONE',  ( 105.0000000000000000, 105.0000000000000568, 240.0000000000000284 ) ) ;
#2285=CARTESIAN_POINT ( 'NONE',  ( 115.0000000000000000, -115.0000000000000000, 270.0000000000000000 ) ) ;
#2290=VECTOR ( 'NONE', #3868, 1000.000000000000000 ) ;
#2297=AXIS2_PLACEMENT_3D ( 'NONE', #1037, #7497, #6690 ) ;
#2299=LINE ( 'NONE', #1061, #98 ) ;
#2301=VECTOR ( 'NONE', #7577, 1000.000000000000000 ) ;
#2305=ORIENTED_EDGE ( 'NONE', *, *, #3755, .F. ) ;
#2312=ORIENTED_EDGE ( 'NONE', *, *, #5305, .T. ) ;
#2319=EDGE_LOOP ( 'NONE', ( #6583, #1120, #8295, #4661 ) ) ;
#2321=LINE ( 'NONE', #2931, #7030 ) ;
#2322=EDGE_CURVE ( 'NONE', #3289, #4789, #5282, .T. ) ;
#2323=EDGE_CURVE ( 'NONE', #6249, #2457, #3389, .T. ) ;
#2326=EDGE_LOOP ( 'NONE', ( #4674, #6501, #5921, #1911 ) ) ;
#2331=ORIENTED_EDGE ( 'NONE', *, *, #2487, .T. ) ;
#2334=DIRECTION ( 'NONE',  ( 0.000000000000000000, 0.000000000000000000, -1.000000000000000000 ) ) ;
#2339=ORIENTED_EDGE ( 'NONE', *, *, #7540, .T. ) ;
#2347=CARTESIAN_POINT ( 'NONE',  ( 125.0000000000000000, 0.000000000000000000, 0.000000000000000000 ) ) ;
#2349=LINE ( 'NONE', #6211, #112 ) ;
#2359=DIRECTION ( 'NONE',  ( -0.000000000000000000, -0.000000000000000000, 1.000000000000000000 ) ) ;
#2365=ORIENTED_EDGE ( 'NONE', *, *, #2427, .F. ) ;
#2366=ADVANCED_FACE ( 'NONE', ( #801 ), #8108, .F. ) ;
#2370=APPLICATION_CONTEXT ( 'automotive_design' ) ;
#2376=EDGE_LOOP ( 'NONE', ( #6968, #5734 ) ) ;
#2393=AXIS2_PLACEMENT_3D ( 'NONE', #3814, #2436, #6465 ) ;
#2397=DIRECTION ( 'NONE',  ( -0.000000000000000000, -0.000000000000000000, 1.000000000000000000 ) ) ;
#2401=DIRECTION ( 'NONE',  ( 0.000000000000000000, -1.000000000000000000, 1.266875999117951024E-16 ) ) ;
#2407=AXIS2_PLACEMENT_3D ( 'NONE', #3647, #6226, #1219 ) ;
#2411=ORIENTED_EDGE ( 'NONE', *, *, #2860, .F. ) ;
#2416=VECTOR ( 'NONE', #4711, 1000.000000000000000 ) ;
#2419=ORIENTED_EDGE ( 'NONE', *, *, #3638, .T. ) ;
#2427=EDGE_CURVE ( 'NONE', #1534, #3826, #1512, .T. ) ;
#2430=EDGE_CURVE ( 'NONE', #509, #6613, #6898, .T. ) ;
#2432=AXIS2_PLACEMENT_3D ( 'NONE', #1469, #102, #7333 ) ;
#2434=CARTESIAN_POINT ( 'NONE',  ( 0.000000000000000000, 125.0000000000000568, 66.99999999999992895 ) ) ;
#2436=DIRECTION ( 'NONE',  ( -0.000000000000000000, -0.000000000000000000, 1.000000000000000000 ) ) ;
#2438=AXIS2_PLACEMENT_3D ( 'NONE', #7024, #1206, #605 ) ;
#2448=ORIENTED_EDGE ( 'NONE', *, *, #3237, .F. ) ;
#2457=VERTEX_POINT ( 'NONE', #355 ) ;
#2458=CARTESIAN_POINT ( 'NONE',  ( -59.99999999999999289, -55.00000000000000000, 220.0000000000000284 ) ) ;
#2461=ORIENTED_EDGE ( 'NONE', *, *, #7161, .F. ) ;
#2468=EDGE_LOOP ( 'NONE', ( #1239, #4779, #1155, #3877, #4051, #5086, #6552, #1588 ) ) ;
#2476=DIRECTION ( 'NONE',  ( 0.000000000000000000, 1.460819769243626884E-16, 1.000000000000000000 ) ) ;
#2485=ADVANCED_FACE ( 'NONE', ( #6057 ), #4862, .F. ) ;
#2487=EDGE_CURVE ( 'NONE', #6953, #3210, #2321, .T. ) ;
#2492=EDGE_LOOP ( 'NONE', ( #7433, #292 ) ) ;
#2493=CARTESIAN_POINT ( 'NONE',  ( 60.00000000000000000, -55.00000000000000000, 240.0000000000000284 ) ) ;
#2496=CARTESIAN_POINT ( 'NONE',  ( -105.0000000000000000, 105.0000000000000853, 20.00000000000000355 ) ) ;
#2503=CARTESIAN_POINT ( 'NONE',  ( 0.000000000000000000, 125.0000000000000568, 66.99999999999992895 ) ) ;
#2518=CARTESIAN_POINT ( 'NONE',  ( -115.0000000000000000, -115.0000000000000000, 270.0000000000000000 ) ) ;
#2527=EDGE_CURVE ( 'NONE', #6613, #509, #7248, .T. ) ;
#2534=LINE ( 'NONE', #2493, #2290 ) ;
#2536=DIRECTION ( 'NONE',  ( -0.8571673007021134438, 1.049727191138620051E-16, 0.5150380749100522682 ) ) ;
#2539=DIRECTION ( 'NONE',  ( 0.8571673007021134438, 0.000000000000000000, 0.5150380749100522682 ) ) ;
#2541=DIRECTION ( 'NONE',  ( 1.000000000000000000, 0.000000000000000000, 0.000000000000000000 ) ) ;
#2542=VECTOR ( 'NONE', #5245, 1000.000000000000000 ) ;
#2543=FACE_OUTER_BOUND ( 'NONE', #4119, .T. ) ;
#2544=VECTOR ( 'NONE', #6864, 1000.000000000000000 ) ;
#2549=CARTESIAN_POINT ( 'NONE',  ( 0.000000000000000000, 52.49999999999997868, 79.99999999999994316 ) ) ;
#2565=CARTESIAN_POINT ( 'NONE',  ( 125.0000000000000000, 52.50000000000000000, 190.0000000000000284 ) ) ;
#2570=VECTOR ( 'NONE', #6633, 1000.000000000000000 ) ;
#2572=VERTEX_POINT ( 'NONE', #6355 ) ;
#2579=ADVANCED_FACE ( 'NONE', ( #3787 ), #7036, .F. ) ;
#2583=CARTESIAN_POINT ( 'NONE',  ( -125.0000000000000000, -52.49999999999997158, 0.000000000000000000 ) ) ;
#2586=ORIENTED_EDGE ( 'NONE', *, *, #510, .T. ) ;
#2587=CARTESIAN_POINT ( 'NONE',  ( 115.0000000000000000, -115.0000000000000000, 270.0000000000000000 ) ) ;
#2594=DIRECTION ( 'NONE',  ( -0.000000000000000000, -0.000000000000000000, 1.000000000000000000 ) ) ;
#2600=ORIENTED_EDGE ( 'NONE', *, *, #7000, .F. ) ;
#2606=DIRECTION ( 'NONE',  ( 1.000000000000000000, 0.000000000000000000, 0.000000000000000000 ) ) ;
#2610=DIRECTION ( 'NONE',  ( -0.000000000000000000, -1.000000000000000000, 1.586032892321652236E-16 ) ) ;
#2614=DIRECTION ( 'NONE',  ( -0.000000000000000000, -1.000000000000000000, 1.586032892321652236E-16 ) ) ;
#2623=LINE ( 'NONE', #1872, #6579 ) ;
#2625=LINE ( 'NONE', #4462, #1809 ) ;
#2630=ADVANCED_FACE ( 'NONE', ( #3143, #7551, #6266, #4265, #489, #4443 ), #3058, .F. ) ;
#2634=DIRECTION ( 'NONE',  ( -0.000000000000000000, -0.000000000000000000, 1.000000000000000000 ) ) ;
#2642=DIRECTION ( 'NONE',  ( -1.000000000000000000, -2.643388153869419325E-16, 0.000000000000000000 ) ) ;
#2653=AXIS2_PLACEMENT_3D ( 'NONE', #7756, #3895, #2476 ) ;
#2654=ORIENTED_EDGE ( 'NONE', *, *, #922, .F. ) ;
#2655=DIRECTION ( 'NONE',  ( -0.000000000000000000, -0.000000000000000000, 1.000000000000000000 ) ) ;
#2658=FACE_OUTER_BOUND ( 'NONE', #4634, .T. ) ;
#2661=ORIENTED_EDGE ( 'NONE', *, *, #2032, .F. ) ;
#2666=CIRCLE ( 'NONE', #7389, 12.99999999999999822 ) ;
#2668=CARTESIAN_POINT ( 'NONE',  ( 50.00000000000000711, 55.00000000000000000, 220.0000000000000284 ) ) ;
#2672=PRODUCT_DEFINITION ( 'UNKNOWN', '', #7994, #233 ) ;
#2691=AXIS2_PLACEMENT_3D ( 'NONE', #5259, #3979, #5333 ) ;
#2695=DIRECTION ( 'NONE',  ( -0.000000000000000000, -0.000000000000000000, 1.000000000000000000 ) ) ;
#2697=CARTESIAN_POINT ( 'NONE',  ( -55.00000000000000000, 55.00000000000000000, 240.0000000000000284 ) ) ;
#2703=FACE_BOUND ( 'NONE', #6143, .T. ) ;
#2708=DIRECTION ( 'NONE',  ( -0.000000000000000000, -0.000000000000000000, 1.000000000000000000 ) ) ;
#2709=CARTESIAN_POINT ( 'NONE',  ( -125.0000000000000000, 52.49999999999997158, 0.000000000000000000 ) ) ;
#2713=ORIENTED_EDGE ( 'NONE', *, *, #397, .T. ) ;
#2714=CARTESIAN_POINT ( 'NONE',  ( -105.0000000000000000, 105.0000000000000284, 240.0000000000000284 ) ) ;
#2716=DIRECTION ( 'NONE',  ( -1.000000000000000000, -0.000000000000000000, -0.000000000000000000 ) ) ;
#2717=CARTESIAN_POINT ( 'NONE',  ( 55.00000000000000000, -55.00000000000000000, 240.0000000000000284 ) ) ;
#2718=( LENGTH_UNIT ( ) NAMED_UNIT ( * ) SI_UNIT ( .MILLI., .METRE. ) );
#2721=ADVANCED_FACE ( 'NONE', ( #746 ), #4484, .F. ) ;
#2732=ORIENTED_EDGE ( 'NONE', *, *, #2279, .T. ) ;
#2740=DIRECTION ( 'NONE',  ( -0.8571673007021116675, 1.049727191138617833E-16, 0.5150380749100552658 ) ) ;
#2742=CARTESIAN_POINT ( 'NONE',  ( -105.0000000000000000, -72.49999999999994316, -212.5000000000000568 ) ) ;
#2745=ORIENTED_EDGE ( 'NONE', *, *, #7529, .T. ) ;
#2747=CONICAL_SURFACE ( 'NONE', #5720, 4.999999999999990230, 1.029744258676653201 ) ;
#2750=AXIS2_PLACEMENT_3D ( 'NONE', #303, #5509, #1628 ) ;
#2755=DIRECTION ( 'NONE',  ( -0.000000000000000000, -0.000000000000000000, 1.000000000000000000 ) ) ;
#2756=PLANE ( 'NONE',  #4396 ) ;
#2758=ORIENTED_EDGE ( 'NONE', *, *, #240, .F. ) ;
#2760=ORIENTED_EDGE ( 'NONE', *, *, #6371, .F. ) ;
#2763=PLANE ( 'NONE',  #4953 ) ;
#2766=CYLINDRICAL_SURFACE ( 'NONE', #2975, 4.999999999999997335 ) ;
#2775=CARTESIAN_POINT ( 'NONE',  ( -50.00000000000000000, 55.00000000000000000, 240.0000000000000284 ) ) ;
#2782=DIRECTION ( 'NONE',  ( 0.000000000000000000, -1.000000000000000000, -1.460819769243626884E-16 ) ) ;
#2783=DIRECTION ( 'NONE',  ( 0.000000000000000000, -1.000000000000000000, -1.266875999117951024E-16 ) ) ;
#2784=CARTESIAN_POINT ( 'NONE',  ( -115.0000000000000000, -115.0000000000000000, 340.0000000000000000 ) ) ;
#2787=CARTESIAN_POINT ( 'NONE',  ( -104.9999999999999432, -105.0000000000000853, 240.0000000000000284 ) ) ;
#2794=VECTOR ( 'NONE', #2594, 1000.000000000000000 ) ;
#2795=CARTESIAN_POINT ( 'NONE',  ( -125.0000000000000000, 52.49999999999997158, 0.000000000000000000 ) ) ;
#2798=ORIENTED_EDGE ( 'NONE', *, *, #240, .T. ) ;
#2825=PLANE ( 'NONE',  #1536 ) ;
#2837=DIRECTION ( 'NONE',  ( 0.8571673007021116675, 0.000000000000000000, 0.5150380749100552658 ) ) ;
#2839=CYLINDRICAL_SURFACE ( 'NONE', #2750, 12.99999999999999822 ) ;
#2843=CARTESIAN_POINT ( 'NONE',  ( 0.000000000000000000, -105.0000000000000711, 66.99999999999997158 ) ) ;
#2846=CARTESIAN_POINT ( 'NONE',  ( 0.000000000000000000, 125.0000000000000568, 66.99999999999992895 ) ) ;
#2857=CARTESIAN_POINT ( 'NONE',  ( -110.0000000000000142, -115.0000000000000000, 340.0000000000000000 ) ) ;
#2858=AXIS2_PLACEMENT_3D ( 'NONE', #247, #544, #4273 ) ;
#2860=EDGE_CURVE ( 'NONE', #3924, #4162, #2014, .T. ) ;
#2862=DIRECTION ( 'NONE',  ( -0.8571673007021134438, 1.049727191138620051E-16, 0.5150380749100522682 ) ) ;
#2864=ORIENTED_EDGE ( 'NONE', *, *, #4321, .F. ) ;
#2866=EDGE_CURVE ( 'NONE', #7449, #5396, #6705, .T. ) ;
#2868=EDGE_CURVE ( 'NONE', #7656, #323, #1547, .T. ) ;
#2869=ORIENTED_EDGE ( 'NONE', *, *, #7051, .F. ) ;
#2870=CYLINDRICAL_SURFACE ( 'NONE', #7663, 4.999999999999990230 ) ;
#2871=DIRECTION ( 'NONE',  ( 1.000000000000000000, -0.000000000000000000, 0.000000000000000000 ) ) ;
#2872=CIRCLE ( 'NONE', #5037, 12.99999999999999822 ) ;
#2880=CARTESIAN_POINT ( 'NONE',  ( 105.0000000000000000, 8.487013464091010249E-14, 20.00000000000001776 ) ) ;
#2882=LINE ( 'NONE', #4145, #4283 ) ;
#2889=ORIENTED_EDGE ( 'NONE', *, *, #4569, .T. ) ;
#2891=ORIENTED_EDGE ( 'NONE', *, *, #8219, .T. ) ;
#2898=CARTESIAN_POINT ( 'NONE',  ( 0.000000000000000000, -52.49999999999996447, 79.99999999999995737 ) ) ;
#2907=ORIENTED_EDGE ( 'NONE', *, *, #4580, .F. ) ;
#2919=CARTESIAN_POINT ( 'NONE',  ( 0.000000000000000000, -72.50000000000000000, 240.0000000000000284 ) ) ;
#2921=DIRECTION ( 'NONE',  ( -0.000000000000000000, -0.000000000000000000, 1.000000000000000000 ) ) ;
#2923=ORIENTED_EDGE ( 'NONE', *, *, #7157, .T. ) ;
#2926=ADVANCED_FACE ( 'NONE', ( #1629, #5970 ), #2756, .T. ) ;
#2931=CARTESIAN_POINT ( 'NONE',  ( -125.0000000000000000, 125.0000000000000000, 340.0000000000000000 ) ) ;
#2934=ORIENTED_EDGE ( 'NONE', *, *, #152, .F. ) ;
#2936=AXIS2_PLACEMENT_3D ( 'NONE', #276, #1141, #5484 ) ;
#2938=EDGE_LOOP ( 'NONE', ( #623, #5176, #3760, #4346 ) ) ;
#2948=VERTEX_POINT ( 'NONE', #5291 ) ;
#2950=VECTOR ( 'NONE', #2716, 1000.000000000000000 ) ;
#2958=CARTESIAN_POINT ( 'NONE',  ( 0.000000000000000000, -105.0000000000000711, 79.99999999999997158 ) ) ;
#2959=ORIENTED_EDGE ( 'NONE', *, *, #1556, .F. ) ;
#2965=LINE ( 'NONE', #4950, #7512 ) ;
#2970=ORIENTED_EDGE ( 'NONE', *, *, #3484, .T. ) ;
#2972=CARTESIAN_POINT ( 'NONE',  ( 60.00000000000000000, 55.00000000000000000, 240.0000000000000284 ) ) ;
#2973=EDGE_LOOP ( 'NONE', ( #424, #2365 ) ) ;
#2975=AXIS2_PLACEMENT_3D ( 'NONE', #2049, #4031, #5898 ) ;
#2982=LINE ( 'NONE', #3658, #2570 ) ;
#2990=FACE_OUTER_BOUND ( 'NONE', #6141, .T. ) ;
#2991=ORIENTED_EDGE ( 'NONE', *, *, #5537, .F. ) ;
#3004=ORIENTED_EDGE ( 'NONE', *, *, #5828, .T. ) ;
#3009=ORIENTED_EDGE ( 'NONE', *, *, #1556, .T. ) ;
#3012=ADVANCED_FACE ( 'NONE', ( #63 ), #468, .F. ) ;
#3018=CARTESIAN_POINT ( 'NONE',  ( 125.0000000000000000, 125.0000000000000000, 340.0000000000000000 ) ) ;
#3022=EDGE_CURVE ( 'NONE', #6613, #1534, #5582, .T. ) ;
#3023=EDGE_LOOP ( 'NONE', ( #1553, #6192, #1782, #6408 ) ) ;
#3034=DIRECTION ( 'NONE',  ( -0.000000000000000000, -1.000000000000000000, 1.586032892321652236E-16 ) ) ;
#3038=ORIENTED_EDGE ( 'NONE', *, *, #3430, .T. ) ;
#3041=LINE ( 'NONE', #6848, #6424 ) ;
#3043=DIRECTION ( 'NONE',  ( 0.000000000000000000, 1.000000000000000000, 1.224646799147353207E-16 ) ) ;
#3047=AXIS2_PLACEMENT_3D ( 'NONE', #4343, #1251, #7105 ) ;
#3048=EDGE_LOOP ( 'NONE', ( #3831, #2798 ) ) ;
#3053=CONICAL_SURFACE ( 'NONE', #1318, 4.999999999999990230, 1.029744258676656754 ) ;
#3054=ORIENTED_EDGE ( 'NONE', *, *, #2268, .F. ) ;
#3058=PLANE ( 'NONE',  #3876 ) ;
#3059=CIRCLE ( 'NONE', #5079, 4.999999999999990230 ) ;
#3061=VECTOR ( 'NONE', #6083, 1000.000000000000000 ) ;
#3071=VECTOR ( 'NONE', #2695, 1000.000000000000000 ) ;
#3079=EDGE_CURVE ( 'NONE', #5024, #3849, #8246, .T. ) ;
#3086=VECTOR ( 'NONE', #7343, 1000.000000000000000 ) ;
#3092=CIRCLE ( 'NONE', #4565, 4.999999999999997335 ) ;
#3104=CARTESIAN_POINT ( 'NONE',  ( 55.00000000000000000, 55.00000000000000000, 240.0000000000000284 ) ) ;
#3111=ORIENTED_EDGE ( 'NONE', *, *, #792, .F. ) ;
#3114=LINE ( 'NONE', #6361, #660 ) ;
#3122=EDGE_CURVE ( 'NONE', #4494, #3982, #839, .T. ) ;
#3129=CARTESIAN_POINT ( 'NONE',  ( 0.000000000000000000, 72.50000000000000000, -212.5000000000000568 ) ) ;
#3130=EDGE_LOOP ( 'NONE', ( #6272, #6468, #8071, #5191 ) ) ;
#3135=EDGE_CURVE ( 'NONE', #5343, #8276, #787, .T. ) ;
#3141=CARTESIAN_POINT ( 'NONE',  ( 0.000000000000000000, 125.0000000000000568, 79.99999999999992895 ) ) ;
#3143=FACE_BOUND ( 'NONE', #7490, .T. ) ;
#3144=ORIENTED_EDGE ( 'NONE', *, *, #7161, .T. ) ;
#3152=VECTOR ( 'NONE', #4540, 1000.000000000000000 ) ;
#3154=EDGE_CURVE ( 'NONE', #3210, #1562, #6658, .T. ) ;
#3156=DIRECTION ( 'NONE',  ( -0.000000000000000000, 1.266875999117951024E-16, 1.000000000000000000 ) ) ;
#3166=CYLINDRICAL_SURFACE ( 'NONE', #7316, 12.99999999999999822 ) ;
#3172=CARTESIAN_POINT ( 'NONE',  ( 1.592040838891560279E-15, -72.49999999999998579, 92.99999999999995737 ) ) ;
#3175=ADVANCED_FACE ( 'NONE', ( #5273 ), #231, .F. ) ;
#3176=DIRECTION ( 'NONE',  ( 0.000000000000000000, -1.000000000000000000, 1.266875999117951024E-16 ) ) ;
#3180=EDGE_LOOP ( 'NONE', ( #336, #972, #1810, #2891 ) ) ;
#3187=EDGE_CURVE ( 'NONE', #1109, #1665, #184, .T. ) ;
#3188=CARTESIAN_POINT ( 'NONE',  ( 60.00000000000000000, -55.00000000000000000, 240.0000000000000284 ) ) ;
#3189=EDGE_CURVE ( 'NONE', #4072, #3924, #3988, .T. ) ;
#3195=AXIS2_PLACEMENT_3D ( 'NONE', #7885, #2610, #3261 ) ;
#3198=ADVANCED_FACE ( 'NONE', ( #798, #2248 ), #2763, .F. ) ;
#3200=VECTOR ( 'NONE', #1017, 1000.000000000000000 ) ;
#3202=CARTESIAN_POINT ( 'NONE',  ( 125.0000000000000000, -125.0000000000000568, -9.184850993605156622E-15 ) ) ;
#3207=LINE ( 'NONE', #564, #2794 ) ;
#3210=VERTEX_POINT ( 'NONE', #3306 ) ;
#3215=AXIS2_PLACEMENT_3D ( 'NONE', #3104, #2397, #5681 ) ;
#3220=DIRECTION ( 'NONE',  ( -0.000000000000000000, -0.000000000000000000, 1.000000000000000000 ) ) ;
#3226=ORIENTED_EDGE ( 'NONE', *, *, #335, .T. ) ;
#3227=EDGE_LOOP ( 'NONE', ( #3384, #5341, #508, #6780 ) ) ;
#3234=DIRECTION ( 'NONE',  ( 1.000000000000000000, 0.000000000000000000, 0.000000000000000000 ) ) ;
#3235=ADVANCED_FACE ( 'NONE', ( #270 ), #7391, .F. ) ;
#3237=EDGE_CURVE ( 'NONE', #6772, #8146, #4030, .T. ) ;
#3240=CARTESIAN_POINT ( 'NONE',  ( 55.00000000000000000, -55.00000000000000000, 240.0000000000000284 ) ) ;
#3241=ORIENTED_EDGE ( 'NONE', *, *, #6708, .F. ) ;
#3247=CARTESIAN_POINT ( 'NONE',  ( -59.99999999999999289, -55.00000000000000000, 220.0000000000000284 ) ) ;
#3248=DIRECTION ( 'NONE',  ( 0.8571673007021134438, 0.000000000000000000, 0.5150380749100522682 ) ) ;
#3255=VECTOR ( 'NONE', #503, 1000.000000000000000 ) ;
#3261=DIRECTION ( 'NONE',  ( 0.000000000000000000, 0.000000000000000000, -1.000000000000000000 ) ) ;
#3268=DIRECTION ( 'NONE',  ( 1.000000000000000000, 0.000000000000000000, 0.000000000000000000 ) ) ;
#3271=DIRECTION ( 'NONE',  ( -0.000000000000000000, -0.000000000000000000, 1.000000000000000000 ) ) ;
#3289=VERTEX_POINT ( 'NONE', #6774 ) ;
#3290=DIRECTION ( 'NONE',  ( -0.000000000000000000, -0.000000000000000000, 1.000000000000000000 ) ) ;
#3303=AXIS2_PLACEMENT_3D ( 'NONE', #736, #3290, #5959 ) ;
#3306=CARTESIAN_POINT ( 'NONE',  ( -125.0000000000000000, 125.0000000000000000, 340.0000000000000000 ) ) ;
#3309=VERTEX_POINT ( 'NONE', #440 ) ;
#3323=LINE ( 'NONE', #851, #7741 ) ;
#3327=ORIENTED_EDGE ( 'NONE', *, *, #7529, .F. ) ;
#3331=EDGE_CURVE ( 'NONE', #5909, #4789, #8089, .T. ) ;
#3338=LINE ( 'NONE', #1458, #4026 ) ;
#3353=CARTESIAN_POINT ( 'NONE',  ( 125.0000000000000000, 52.49999999999997158, 0.000000000000000000 ) ) ;
#3362=FACE_OUTER_BOUND ( 'NONE', #7700, .T. ) ;
#3364=CARTESIAN_POINT ( 'NONE',  ( 125.0000000000000000, -52.49999999999997158, 0.000000000000000000 ) ) ;
#3384=ORIENTED_EDGE ( 'NONE', *, *, #131, .T. ) ;
#3389=LINE ( 'NONE', #7859, #1107 ) ;
#3395=VECTOR ( 'NONE', #2862, 1000.000000000000000 ) ;
#3397=CARTESIAN_POINT ( 'NONE',  ( 125.0000000000000000, -125.0000000000000568, -9.184850993605156622E-15 ) ) ;
#3406=VERTEX_POINT ( 'NONE', #1379 ) ;
#3412=CARTESIAN_POINT ( 'NONE',  ( 50.00000000000000711, -55.00000000000000000, 220.0000000000000284 ) ) ;
#3421=LINE ( 'NONE', #17, #3467 ) ;
#3427=DIRECTION ( 'NONE',  ( 1.000000000000000000, 0.000000000000000000, 0.000000000000000000 ) ) ;
#3430=EDGE_CURVE ( 'NONE', #5443, #7579, #2127, .T. ) ;
#3431=AXIS2_PLACEMENT_3D ( 'NONE', #1218, #7805, #6389 ) ;
#3437=CARTESIAN_POINT ( 'NONE',  ( 0.000000000000000000, 105.0000000000000426, 79.99999999999992895 ) ) ;
#3444=FACE_BOUND ( 'NONE', #2376, .T. ) ;
#3448=ORIENTED_EDGE ( 'NONE', *, *, #7106, .F. ) ;
#3450=DIRECTION ( 'NONE',  ( -0.000000000000000000, -0.000000000000000000, 1.000000000000000000 ) ) ;
#3462=CARTESIAN_POINT ( 'NONE',  ( -60.00000000000000000, -55.00000000000000000, 240.0000000000000284 ) ) ;
#3464=FACE_OUTER_BOUND ( 'NONE', #3951, .T. ) ;
#3467=VECTOR ( 'NONE', #2614, 1000.000000000000000 ) ;
#3478=VERTEX_POINT ( 'NONE', #136 ) ;
#3482=EDGE_CURVE ( 'NONE', #1112, #4879, #7096, .T. ) ;
#3484=EDGE_CURVE ( 'NONE', #4695, #8274, #1544, .T. ) ;
#3487=EDGE_LOOP ( 'NONE', ( #6187, #3448, #4579, #1038 ) ) ;
#3490=DIRECTION ( 'NONE',  ( -1.000000000000000000, 0.000000000000000000, -0.000000000000000000 ) ) ;
#3491=LINE ( 'NONE', #2742, #5923 ) ;
#3498=VECTOR ( 'NONE', #5612, 1000.000000000000000 ) ;
#3500=DIRECTION ( 'NONE',  ( -0.000000000000000000, -0.000000000000000000, 1.000000000000000000 ) ) ;
#3504=CARTESIAN_POINT ( 'NONE',  ( -120.0000000000000000, -115.0000000000000000, 270.0000000000000000 ) ) ;
#3507=CYLINDRICAL_SURFACE ( 'NONE', #7407, 4.999999999999997335 ) ;
#3515=CARTESIAN_POINT ( 'NONE',  ( 105.0000000000000000, 105.0000000000000853, 20.00000000000000355 ) ) ;
#3529=CARTESIAN_POINT ( 'NONE',  ( -115.0000000000000142, -115.0000000000000000, 266.9956969048622568 ) ) ;
#3536=PLANE ( 'NONE',  #1480 ) ;
#3542=DIRECTION ( 'NONE',  ( -0.000000000000000000, -0.000000000000000000, 1.000000000000000000 ) ) ;
#3545=CIRCLE ( 'NONE', #5725, 4.999999999999990230 ) ;
#3549=EDGE_CURVE ( 'NONE', #5775, #3690, #5802, .T. ) ;
#3551=EDGE_LOOP ( 'NONE', ( #6996, #6319, #1710 ) ) ;
#3554=ORIENTED_EDGE ( 'NONE', *, *, #792, .T. ) ;
#3562=ORIENTED_EDGE ( 'NONE', *, *, #5168, .F. ) ;
#3568=CARTESIAN_POINT ( 'NONE',  ( 114.9999999999999858, 115.0000000000000000, 266.9956969048622568 ) ) ;
#3569=CONICAL_SURFACE ( 'NONE', #3303, 4.999999999999990230, 1.029744258676653201 ) ;
#3571=ORIENTED_EDGE ( 'NONE', *, *, #4825, .F. ) ;
#3572=EDGE_CURVE ( 'NONE', #7416, #1211, #4790, .T. ) ;
#3574=ADVANCED_FACE ( 'NONE', ( #7670, #3850 ), #5715, .F. ) ;
#3579=DIRECTION ( 'NONE',  ( -1.000000000000000000, -0.000000000000000000, 0.000000000000000000 ) ) ;
#3585=EDGE_CURVE ( 'NONE', #4085, #5646, #7504, .T. ) ;
#3586=ADVANCED_FACE ( 'NONE', ( #1326 ), #7232, .F. ) ;
#3589=EDGE_LOOP ( 'NONE', ( #7295, #3674, #4461, #6883 ) ) ;
#3606=ORIENTED_EDGE ( 'NONE', *, *, #4699, .F. ) ;
#3607=DIRECTION ( 'NONE',  ( 0.000000000000000000, 0.000000000000000000, -1.000000000000000000 ) ) ;
#3608=DIRECTION ( 'NONE',  ( 0.000000000000000000, -1.000000000000000000, 1.266875999117951024E-16 ) ) ;
#3610=ORIENTED_EDGE ( 'NONE', *, *, #2322, .F. ) ;
#3615=CARTESIAN_POINT ( 'NONE',  ( 105.0000000000000000, 72.50000000000000000, -212.5000000000000568 ) ) ;
#3626=CARTESIAN_POINT ( 'NONE',  ( 125.0000000000000000, -52.49999999999997158, 0.000000000000000000 ) ) ;
#3638=EDGE_CURVE ( 'NONE', #8274, #1093, #7147, .T. ) ;
#3641=EDGE_CURVE ( 'NONE', #3478, #1112, #7228, .T. ) ;
#3643=DIRECTION ( 'NONE',  ( -0.000000000000000000, -1.000000000000000000, 1.586032892321652236E-16 ) ) ;
#3647=CARTESIAN_POINT ( 'NONE',  ( -55.00000000000000000, 55.00000000000000000, 240.0000000000000284 ) ) ;
#3650=ORIENTED_EDGE ( 'NONE', *, *, #871, .F. ) ;
#3652=DIRECTION ( 'NONE',  ( -1.000000000000000000, -0.000000000000000000, -0.000000000000000000 ) ) ;
#3657=DIRECTION ( 'NONE',  ( -0.000000000000000000, -1.000000000000000000, 1.586032892321652236E-16 ) ) ;
#3658=CARTESIAN_POINT ( 'NONE',  ( -110.0000000000000142, 115.0000000000000000, 340.0000000000000000 ) ) ;
#3662=CARTESIAN_POINT ( 'NONE',  ( 0.000000000000000000, -105.0000000000000568, 20.00000000000001776 ) ) ;
#3674=ORIENTED_EDGE ( 'NONE', *, *, #5796, .T. ) ;
#3680=AXIS2_PLACEMENT_3D ( 'NONE', #3364, #8023, #2783 ) ;
#3689=ADVANCED_FACE ( 'NONE', ( #4690 ), #3569, .F. ) ;
#3690=VERTEX_POINT ( 'NONE', #2067 ) ;
#3694=VECTOR ( 'NONE', #4751, 1000.000000000000000 ) ;
#3695=ADVANCED_FACE ( 'NONE', ( #5877 ), #7951, .F. ) ;
#3710=FACE_OUTER_BOUND ( 'NONE', #7799, .T. ) ;
#3714=DIRECTION ( 'NONE',  ( -0.000000000000000000, -1.000000000000000000, 1.586032892321652236E-16 ) ) ;
#3718=EDGE_LOOP ( 'NONE', ( #5371, #5760, #223, #2923 ) ) ;
#3719=ORIENTED_EDGE ( 'NONE', *, *, #3585, .T. ) ;
#3722=FACE_OUTER_BOUND ( 'NONE', #5739, .T. ) ;
#3724=LINE ( 'NONE', #5676, #4154 ) ;
#3730=EDGE_LOOP ( 'NONE', ( #6661, #2654, #1997, #648 ) ) ;
#3749=AXIS2_PLACEMENT_3D ( 'NONE', #3, #1929, #5027 ) ;
#3753=ORIENTED_EDGE ( 'NONE', *, *, #3755, .T. ) ;
#3755=EDGE_CURVE ( 'NONE', #6237, #5271, #5320, .T. ) ;
#3758=ORIENTED_EDGE ( 'NONE', *, *, #4437, .T. ) ;
#3759=LINE ( 'NONE', #2503, #2144 ) ;
#3760=ORIENTED_EDGE ( 'NONE', *, *, #2427, .T. ) ;
#3768=VERTEX_POINT ( 'NONE', #279 ) ;
#3770=ORIENTED_EDGE ( 'NONE', *, *, #1643, .T. ) ;
#3775=ORIENTED_EDGE ( 'NONE', *, *, #5168, .T. ) ;
#3781=DIRECTION ( 'NONE',  ( -0.000000000000000000, -1.000000000000000000, 1.586032892321652236E-16 ) ) ;
#3783=CARTESIAN_POINT ( 'NONE',  ( 125.0000000000000000, -52.49999999999997158, 0.000000000000000000 ) ) ;
#3786=PRODUCT_DEFINITION_SHAPE ( 'NONE', 'NONE',  #2672 ) ;
#3787=FACE_OUTER_BOUND ( 'NONE', #3730, .T. ) ;
#3793=ORIENTED_EDGE ( 'NONE', *, *, #309, .T. ) ;
#3797=AXIS2_PLACEMENT_3D ( 'NONE', #4538, #187, #754 ) ;
#3800=ORIENTED_EDGE ( 'NONE', *, *, #7797, .T. ) ;
#3810=LINE ( 'NONE', #3247, #7383 ) ;
#3814=CARTESIAN_POINT ( 'NONE',  ( -55.00000000000000000, 55.00000000000000000, 220.0000000000000284 ) ) ;
#3818=ADVANCED_FACE ( 'NONE', ( #5652 ), #4798, .F. ) ;
#3826=VERTEX_POINT ( 'NONE', #1819 ) ;
#3831=ORIENTED_EDGE ( 'NONE', *, *, #6013, .T. ) ;
#3837=VERTEX_POINT ( 'NONE', #3018 ) ;
#3841=DIRECTION ( 'NONE',  ( -0.000000000000000000, -0.000000000000000000, 1.000000000000000000 ) ) ;
#3845=LINE ( 'NONE', #5797, #6303 ) ;
#3847=FACE_BOUND ( 'NONE', #1243, .T. ) ;
#3848=EDGE_CURVE ( 'NONE', #6212, #416, #5486, .T. ) ;
#3849=VERTEX_POINT ( 'NONE', #1212 ) ;
#3850=FACE_OUTER_BOUND ( 'NONE', #346, .T. ) ;
#3854=ORIENTED_EDGE ( 'NONE', *, *, #5451, .T. ) ;
#3868=DIRECTION ( 'NONE',  ( -0.000000000000000000, -0.000000000000000000, 1.000000000000000000 ) ) ;
#3870=ORIENTED_EDGE ( 'NONE', *, *, #2487, .F. ) ;
#3872=CARTESIAN_POINT ( 'NONE',  ( 110.0000000000000142, -115.0000000000000000, 340.0000000000000000 ) ) ;
#3874=LINE ( 'NONE', #1954, #260 ) ;
#3876=AXIS2_PLACEMENT_3D ( 'NONE', #5645, #8270, #622 ) ;
#3877=ORIENTED_EDGE ( 'NONE', *, *, #6123, .T. ) ;
#3879=DIRECTION ( 'NONE',  ( 0.000000000000000000, 0.000000000000000000, -1.000000000000000000 ) ) ;
#3895=DIRECTION ( 'NONE',  ( 0.000000000000000000, 1.000000000000000000, -1.460819769243626884E-16 ) ) ;
#3902=CARTESIAN_POINT ( 'NONE',  ( -115.0000000000000000, -115.0000000000000000, 270.0000000000000000 ) ) ;
#3914=VECTOR ( 'NONE', #1649, 1000.000000000000000 ) ;
#3920=EDGE_CURVE ( 'NONE', #8240, #4180, #4345, .T. ) ;
#3923=FACE_OUTER_BOUND ( 'NONE', #3487, .T. ) ;
#3924=VERTEX_POINT ( 'NONE', #889 ) ;
#3931=CARTESIAN_POINT ( 'NONE',  ( 115.0000000000000000, 115.0000000000000000, 270.0000000000000000 ) ) ;
#3932=DIRECTION ( 'NONE',  ( 0.000000000000000000, 1.000000000000000000, -1.460819769243626884E-16 ) ) ;
#3933=DIRECTION ( 'NONE',  ( 0.000000000000000000, 0.000000000000000000, -1.000000000000000000 ) ) ;
#3939=CARTESIAN_POINT ( 'NONE',  ( 1.592040838891559490E-15, 125.0000000000000568, 92.99999999999992895 ) ) ;
#3942=( NAMED_UNIT ( * ) PLANE_ANGLE_UNIT ( ) SI_UNIT ( $, .RADIAN. ) );
#3951=EDGE_LOOP ( 'NONE', ( #2661, #1232, #5887 ) ) ;
#3952=CARTESIAN_POINT ( 'NONE',  ( -120.0000000000000000, 115.0000000000000000, 340.0000000000000000 ) ) ;
#3960=AXIS2_PLACEMENT_3D ( 'NONE', #3977, #782, #7881 ) ;
#3971=DIRECTION ( 'NONE',  ( 0.000000000000000000, -1.000000000000000000, 1.586032892321652236E-16 ) ) ;
#3977=CARTESIAN_POINT ( 'NONE',  ( 55.00000000000000000, -55.00000000000000000, 220.0000000000000284 ) ) ;
#3979=DIRECTION ( 'NONE',  ( -0.000000000000000000, -0.000000000000000000, 1.000000000000000000 ) ) ;
#3980=AXIS2_PLACEMENT_3D ( 'NONE', #7921, #2755, #7997 ) ;
#3982=VERTEX_POINT ( 'NONE', #4866 ) ;
#3987=CARTESIAN_POINT ( 'NONE',  ( -55.00000000000000000, -55.00000000000000000, 240.0000000000000284 ) ) ;
#3988=LINE ( 'NONE', #2846, #5362 ) ;
#3989=LINE ( 'NONE', #3353, #5140 ) ;
#3994=CONICAL_SURFACE ( 'NONE', #219, 4.999999999999990230, 1.029744258676653201 ) ;
#4005=DIRECTION ( 'NONE',  ( -0.000000000000000000, -0.000000000000000000, 1.000000000000000000 ) ) ;
#4013=DIRECTION ( 'NONE',  ( -0.000000000000000000, -0.000000000000000000, 1.000000000000000000 ) ) ;
#4017=LINE ( 'NONE', #2074, #2950 ) ;
#4019=VECTOR ( 'NONE', #6055, 1000.000000000000000 ) ;
#4026=VECTOR ( 'NONE', #93, 1000.000000000000000 ) ;
#4030=LINE ( 'NONE', #5003, #2544 ) ;
#4031=DIRECTION ( 'NONE',  ( -0.000000000000000000, -0.000000000000000000, 1.000000000000000000 ) ) ;
#4046=CARTESIAN_POINT ( 'NONE',  ( 115.0000000000000000, 115.0000000000000000, 340.0000000000000000 ) ) ;
#4049=EDGE_CURVE ( 'NONE', #7975, #6953, #2965, .T. ) ;
#4051=ORIENTED_EDGE ( 'NONE', *, *, #3638, .F. ) ;
#4053=FACE_BOUND ( 'NONE', #2051, .T. ) ;
#4062=ORIENTED_EDGE ( 'NONE', *, *, #5426, .F. ) ;
#4072=VERTEX_POINT ( 'NONE', #5596 ) ;
#4078=DIRECTION ( 'NONE',  ( 0.000000000000000000, 1.632680918566406547E-16, -1.000000000000000000 ) ) ;
#4082=FACE_BOUND ( 'NONE', #6380, .T. ) ;
#4085=VERTEX_POINT ( 'NONE', #8262 ) ;
#4088=ORIENTED_EDGE ( 'NONE', *, *, #2172, .F. ) ;
#4096=DIRECTION ( 'NONE',  ( 0.000000000000000000, 0.000000000000000000, -1.000000000000000000 ) ) ;
#4110=EDGE_LOOP ( 'NONE', ( #4975, #3111, #2600, #1062, #5216, #6224, #7734, #1974 ) ) ;
#4113=ORIENTED_EDGE ( 'NONE', *, *, #1647, .F. ) ;
#4114=CARTESIAN_POINT ( 'NONE',  ( 0.000000000000000000, 105.0000000000000426, 66.99999999999992895 ) ) ;
#4119=EDGE_LOOP ( 'NONE', ( #2934, #4793, #6479 ) ) ;
#4120=LINE ( 'NONE', #6150, #2190 ) ;
#4122=EDGE_CURVE ( 'NONE', #5539, #6702, #6148, .T. ) ;
#4124=AXIS2_PLACEMENT_3D ( 'NONE', #6919, #6956, #1095 ) ;
#4125=CARTESIAN_POINT ( 'NONE',  ( 0.000000000000000000, 0.000000000000000000, 240.0000000000000284 ) ) ;
#4130=VECTOR ( 'NONE', #7929, 1000.000000000000000 ) ;
#4135=ORIENTED_EDGE ( 'NONE', *, *, #1806, .T. ) ;
#4138=CYLINDRICAL_SURFACE ( 'NONE', #3980, 4.999999999999990230 ) ;
#4140=ORIENTED_EDGE ( 'NONE', *, *, #6373, .F. ) ;
#4145=CARTESIAN_POINT ( 'NONE',  ( -125.0000000000000000, 52.50000000000000000, 190.0000000000000284 ) ) ;
#4150=DIRECTION ( 'NONE',  ( -0.000000000000000000, -0.000000000000000000, 1.000000000000000000 ) ) ;
#4154=VECTOR ( 'NONE', #8253, 1000.000000000000000 ) ;
#4162=VERTEX_POINT ( 'NONE', #3172 ) ;
#4163=DIRECTION ( 'NONE',  ( -0.000000000000000000, 1.000000000000000000, 1.224646799147353207E-16 ) ) ;
#4164=EDGE_CURVE ( 'NONE', #3309, #4162, #7111, .T. ) ;
#4170=ADVANCED_FACE ( 'NONE', ( #6349 ), #3053, .F. ) ;
#4180=VERTEX_POINT ( 'NONE', #2072 ) ;
#4181=FACE_OUTER_BOUND ( 'NONE', #6935, .T. ) ;
#4185=ORIENTED_EDGE ( 'NONE', *, *, #922, .T. ) ;
#4189=ORIENTED_EDGE ( 'NONE', *, *, #7897, .F. ) ;
#4193=CARTESIAN_POINT ( 'NONE',  ( 110.0000000000000142, -115.0000000000000000, 270.0000000000000000 ) ) ;
#4203=VECTOR ( 'NONE', #2740, 1000.000000000000000 ) ;
#4244=ORIENTED_EDGE ( 'NONE', *, *, #7362, .T. ) ;
#4265=FACE_BOUND ( 'NONE', #2973, .T. ) ;
#4272=AXIS2_PLACEMENT_3D ( 'NONE', #4843, #3657, #3607 ) ;
#4273=DIRECTION ( 'NONE',  ( 1.000000000000000000, 0.000000000000000000, 0.000000000000000000 ) ) ;
#4281=ORIENTED_EDGE ( 'NONE', *, *, #7807, .T. ) ;
#4283=VECTOR ( 'NONE', #6739, 1000.000000000000000 ) ;
#4293=CARTESIAN_POINT ( 'NONE',  ( 55.00000000000000000, 55.00000000000000000, 220.0000000000000284 ) ) ;
#4315=EDGE_LOOP ( 'NONE', ( #2713, #1032, #2461, #6410 ) ) ;
#4317=DIRECTION ( 'NONE',  ( 0.000000000000000000, -1.000000000000000000, 1.586032892321652236E-16 ) ) ;
#4320=FACE_OUTER_BOUND ( 'NONE', #6679, .T. ) ;
#4321=EDGE_CURVE ( 'NONE', #1665, #5271, #3059, .T. ) ;
#4322=ADVANCED_FACE ( 'NONE', ( #903, #4053 ), #297, .F. ) ;
#4330=LINE ( 'NONE', #3615, #3200 ) ;
#4343=CARTESIAN_POINT ( 'NONE',  ( 0.000000000000000000, 125.0000000000000568, 79.99999999999992895 ) ) ;
#4345=LINE ( 'NONE', #333, #7920 ) ;
#4346=ORIENTED_EDGE ( 'NONE', *, *, #5085, .F. ) ;
#4357=ADVANCED_FACE ( 'NONE', ( #6641 ), #2870, .F. ) ;
#4361=CARTESIAN_POINT ( 'NONE',  ( -59.99999999999999289, 55.00000000000000000, 220.0000000000000284 ) ) ;
#4380=EDGE_LOOP ( 'NONE', ( #5714, #452, #5454 ) ) ;
#4385=CARTESIAN_POINT ( 'NONE',  ( 105.0000000000000000, -105.0000000000000568, 20.00000000000001776 ) ) ;
#4396=AXIS2_PLACEMENT_3D ( 'NONE', #1972, #5956, #164 ) ;
#4404=ADVANCED_FACE ( 'NONE', ( #7193 ), #3994, .F. ) ;
#4410=FACE_OUTER_BOUND ( 'NONE', #3718, .T. ) ;
#4414=DIRECTION ( 'NONE',  ( -0.000000000000000000, -1.632680918566406547E-16, 1.000000000000000000 ) ) ;
#4416=DIRECTION ( 'NONE',  ( -0.000000000000000000, -0.000000000000000000, 1.000000000000000000 ) ) ;
#4418=EDGE_LOOP ( 'NONE', ( #4436, #4827, #2732, #6248 ) ) ;
#4421=AXIS2_PLACEMENT_3D ( 'NONE', #174, #6645, #5846 ) ;
#4424=CARTESIAN_POINT ( 'NONE',  ( -105.0000000000000000, -72.50000000000000000, 240.0000000000000284 ) ) ;
#4436=ORIENTED_EDGE ( 'NONE', *, *, #1357, .F. ) ;
#4437=EDGE_CURVE ( 'NONE', #1562, #2572, #3041, .T. ) ;
#4443=FACE_OUTER_BOUND ( 'NONE', #5398, .T. ) ;
#4454=AXIS2_PLACEMENT_3D ( 'NONE', #7895, #1391, #6532 ) ;
#4461=ORIENTED_EDGE ( 'NONE', *, *, #2866, .T. ) ;
#4462=CARTESIAN_POINT ( 'NONE',  ( 50.00000000000000000, -55.00000000000000000, 240.0000000000000284 ) ) ;
#4464=ORIENTED_EDGE ( 'NONE', *, *, #1759, .F. ) ;
#4471=CARTESIAN_POINT ( 'NONE',  ( 0.000000000000000000, 125.0000000000000568, 66.99999999999992895 ) ) ;
#4475=CARTESIAN_POINT ( 'NONE',  ( 55.00000000000000000, -55.00000000000000000, 220.0000000000000284 ) ) ;
#4477=DIRECTION ( 'NONE',  ( -0.000000000000000000, -0.000000000000000000, 1.000000000000000000 ) ) ;
#4479=DIRECTION ( 'NONE',  ( -0.000000000000000000, 1.000000000000000000, 1.266875999117951024E-16 ) ) ;
#4484=CYLINDRICAL_SURFACE ( 'NONE', #3195, 12.99999999999999822 ) ;
#4490=CARTESIAN_POINT ( 'NONE',  ( 114.9999999999999858, -115.0000000000000000, 266.9956969048622568 ) ) ;
#4494=VERTEX_POINT ( 'NONE', #6892 ) ;
#4496=ORIENTED_EDGE ( 'NONE', *, *, #2866, .F. ) ;
#4513=ADVANCED_FACE ( 'NONE', ( #1658 ), #1029, .F. ) ;
#4518=LINE ( 'NONE', #7152, #4639 ) ;
#4532=CARTESIAN_POINT ( 'NONE',  ( -115.0000000000000000, -115.0000000000000000, 270.0000000000000000 ) ) ;
#4536=EDGE_CURVE ( 'NONE', #5024, #3768, #5230, .T. ) ;
#4537=AXIS2_PLACEMENT_3D ( 'NONE', #2347, #3579, #5545 ) ;
#4538=CARTESIAN_POINT ( 'NONE',  ( 55.00000000000000000, 55.00000000000000000, 240.0000000000000284 ) ) ;
#4540=DIRECTION ( 'NONE',  ( -0.000000000000000000, 1.000000000000000000, 1.266875999117951024E-16 ) ) ;
#4554=CIRCLE ( 'NONE', #1604, 4.999999999999990230 ) ;
#4559=ORIENTED_EDGE ( 'NONE', *, *, #4321, .T. ) ;
#4563=EDGE_CURVE ( 'NONE', #6237, #1109, #6704, .T. ) ;
#4564=AXIS2_PLACEMENT_3D ( 'NONE', #1088, #3643, #6222 ) ;
#4565=AXIS2_PLACEMENT_3D ( 'NONE', #1323, #2634, #6463 ) ;
#4567=FACE_OUTER_BOUND ( 'NONE', #2199, .T. ) ;
#4569=EDGE_CURVE ( 'NONE', #4494, #8125, #3845, .T. ) ;
#4571=DIRECTION ( 'NONE',  ( 2.643388153869419325E-16, -1.000000000000000000, 0.000000000000000000 ) ) ;
#4573=AXIS2_PLACEMENT_3D ( 'NONE', #2958, #5377, #5546 ) ;
#4577=EDGE_CURVE ( 'NONE', #2109, #5395, #2666, .T. ) ;
#4579=ORIENTED_EDGE ( 'NONE', *, *, #8053, .T. ) ;
#4580=EDGE_CURVE ( 'NONE', #1935, #6702, #3810, .T. ) ;
#4584=ADVANCED_FACE ( 'NONE', ( #1839 ), #6504, .F. ) ;
#4587=CARTESIAN_POINT ( 'NONE',  ( 0.000000000000000000, 125.0000000000000568, 79.99999999999992895 ) ) ;
#4597=DIRECTION ( 'NONE',  ( -0.000000000000000000, -0.000000000000000000, 1.000000000000000000 ) ) ;
#4598=CARTESIAN_POINT ( 'NONE',  ( 125.0000000000000000, 125.0000000000000000, 340.0000000000000000 ) ) ;
#4603=CYLINDRICAL_SURFACE ( 'NONE', #3215, 4.999999999999997335 ) ;
#4612=PLANE ( 'NONE',  #6188 ) ;
#4627=FACE_OUTER_BOUND ( 'NONE', #962, .T. ) ;
#4632=AXIS2_PLACEMENT_3D ( 'NONE', #2549, #1070, #728 ) ;
#4634=EDGE_LOOP ( 'NONE', ( #2182, #7769, #1195, #2991 ) ) ;
#4635=LINE ( 'NONE', #2583, #3152 ) ;
#4638=( LENGTH_UNIT ( ) NAMED_UNIT ( * ) SI_UNIT ( .MILLI., .METRE. ) );
#4639=VECTOR ( 'NONE', #5963, 1000.000000000000000 ) ;
#4642=EDGE_CURVE ( 'NONE', #3406, #8276, #3207, .T. ) ;
#4659=CIRCLE ( 'NONE', #3431, 4.999999999999990230 ) ;
#4661=ORIENTED_EDGE ( 'NONE', *, *, #8053, .F. ) ;
#4672=EDGE_LOOP ( 'NONE', ( #1044, #2745, #4185 ) ) ;
#4674=ORIENTED_EDGE ( 'NONE', *, *, #5736, .F. ) ;
#4680=CARTESIAN_POINT ( 'NONE',  ( 105.0000000000000000, -105.0000000000000568, 340.0000000000000000 ) ) ;
#4683=VECTOR ( 'NONE', #3034, 1000.000000000000000 ) ;
#4690=FACE_OUTER_BOUND ( 'NONE', #4930, .T. ) ;
#4691=VECTOR ( 'NONE', #2254, 1000.000000000000000 ) ;
#4695=VERTEX_POINT ( 'NONE', #2012 ) ;
#4699=EDGE_CURVE ( 'NONE', #3768, #6134, #603, .T. ) ;
#4702=AXIS2_PLACEMENT_3D ( 'NONE', #7630, #5808, #5125 ) ;
#4704=DIRECTION ( 'NONE',  ( 1.000000000000000000, 0.000000000000000000, 0.000000000000000000 ) ) ;
#4710=DIRECTION ( 'NONE',  ( -0.000000000000000000, -1.000000000000000000, 1.586032892321652236E-16 ) ) ;
#4711=DIRECTION ( 'NONE',  ( -0.000000000000000000, -1.000000000000000000, -0.000000000000000000 ) ) ;
#4713=CARTESIAN_POINT ( 'NONE',  ( 115.0000000000000000, -115.0000000000000000, 340.0000000000000000 ) ) ;
#4719=CARTESIAN_POINT ( 'NONE',  ( 125.0000000000000000, -125.0000000000000000, 340.0000000000000000 ) ) ;
#4722=CARTESIAN_POINT ( 'NONE',  ( -125.0000000000000000, 125.0000000000000568, -9.184850993605156622E-15 ) ) ;
#4723=CARTESIAN_POINT ( 'NONE',  ( 55.00000000000000000, 55.00000000000000000, 240.0000000000000284 ) ) ;
#4724=DIRECTION ( 'NONE',  ( -0.000000000000000000, 1.000000000000000000, 1.224646799147353207E-16 ) ) ;
#4731=AXIS2_PLACEMENT_3D ( 'NONE', #2285, #4788, #4752 ) ;
#4732=ADVANCED_FACE ( 'NONE', ( #3362 ), #7221, .F. ) ;
#4736=CARTESIAN_POINT ( 'NONE',  ( 115.0000000000000000, -115.0000000000000000, 340.0000000000000000 ) ) ;
#4740=DIRECTION ( 'NONE',  ( -0.000000000000000000, -0.000000000000000000, 1.000000000000000000 ) ) ;
#4747=DIRECTION ( 'NONE',  ( 0.000000000000000000, 1.000000000000000000, -1.266875999117951024E-16 ) ) ;
#4751=DIRECTION ( 'NONE',  ( -0.000000000000000000, -0.000000000000000000, 1.000000000000000000 ) ) ;
#4752=DIRECTION ( 'NONE',  ( 1.000000000000000000, 0.000000000000000000, 0.000000000000000000 ) ) ;
#4756=CARTESIAN_POINT ( 'NONE',  ( 105.0000000000000000, -105.0000000000000568, 340.0000000000000000 ) ) ;
#4772=CARTESIAN_POINT ( 'NONE',  ( 50.00000000000000000, -55.00000000000000000, 240.0000000000000284 ) ) ;
#4779=ORIENTED_EDGE ( 'NONE', *, *, #8140, .F. ) ;
#4786=CARTESIAN_POINT ( 'NONE',  ( 120.0000000000000000, 115.0000000000000000, 340.0000000000000000 ) ) ;
#4788=DIRECTION ( 'NONE',  ( -0.000000000000000000, -0.000000000000000000, 1.000000000000000000 ) ) ;
#4789=VERTEX_POINT ( 'NONE', #2173 ) ;
#4790=CIRCLE ( 'NONE', #1033, 4.999999999999990230 ) ;
#4793=ORIENTED_EDGE ( 'NONE', *, *, #2164, .T. ) ;
#4798=CONICAL_SURFACE ( 'NONE', #4124, 4.999999999999990230, 1.029744258676656754 ) ;
#4799=ORIENTED_EDGE ( 'NONE', *, *, #2172, .T. ) ;
#4802=DIRECTION ( 'NONE',  ( -0.000000000000000000, -0.000000000000000000, 1.000000000000000000 ) ) ;
#4815=AXIS2_PLACEMENT_3D ( 'NONE', #6335, #553, #2541 ) ;
#4820=AXIS2_PLACEMENT_3D ( 'NONE', #4598, #810, #4078 ) ;
#4824=AXIS2_PLACEMENT_3D ( 'NONE', #5983, #1395, #149 ) ;
#4825=EDGE_CURVE ( 'NONE', #1918, #717, #5910, .T. ) ;
#4827=ORIENTED_EDGE ( 'NONE', *, *, #4642, .T. ) ;
#4836=EDGE_CURVE ( 'NONE', #67, #448, #78, .T. ) ;
#4841=CARTESIAN_POINT ( 'NONE',  ( 1.592040838891560279E-15, -105.0000000000000711, 92.99999999999997158 ) ) ;
#4843=CARTESIAN_POINT ( 'NONE',  ( 0.000000000000000000, 125.0000000000000568, 79.99999999999992895 ) ) ;
#4848=EDGE_CURVE ( 'NONE', #8106, #4695, #4330, .T. ) ;
#4850=DIRECTION ( 'NONE',  ( 0.000000000000000000, -1.000000000000000000, 1.266875999117951024E-16 ) ) ;
#4862=CONICAL_SURFACE ( 'NONE', #1786, 4.999999999999990230, 1.029744258676656754 ) ;
#4866=CARTESIAN_POINT ( 'NONE',  ( 105.0000000000000000, -72.50000000000001421, 240.0000000000000284 ) ) ;
#4867=CARTESIAN_POINT ( 'NONE',  ( 59.99999999999999289, 55.00000000000000000, 220.0000000000000284 ) ) ;
#4870=DIRECTION ( 'NONE',  ( -0.000000000000000000, -0.000000000000000000, 1.000000000000000000 ) ) ;
#4879=VERTEX_POINT ( 'NONE', #6242 ) ;
#4893=LINE ( 'NONE', #6835, #3255 ) ;
#4896=CIRCLE ( 'NONE', #6171, 12.99999999999999822 ) ;
#4903=ORIENTED_EDGE ( 'NONE', *, *, #3331, .F. ) ;
#4910=CARTESIAN_POINT ( 'NONE',  ( -55.00000000000000000, -55.00000000000000000, 240.0000000000000284 ) ) ;
#4930=EDGE_LOOP ( 'NONE', ( #1383, #2156, #4281 ) ) ;
#4937=ORIENTED_EDGE ( 'NONE', *, *, #1098, .F. ) ;
#4950=CARTESIAN_POINT ( 'NONE',  ( 125.0000000000000000, 125.0000000000000568, -9.184850993605156622E-15 ) ) ;
#4953=AXIS2_PLACEMENT_3D ( 'NONE', #7969, #2203, #5345 ) ;
#4955=LINE ( 'NONE', #6693, #4019 ) ;
#4962=ORIENTED_EDGE ( 'NONE', *, *, #3079, .F. ) ;
#4972=CONICAL_SURFACE ( 'NONE', #8073, 4.999999999999990230, 1.029744258676656754 ) ;
#4975=ORIENTED_EDGE ( 'NONE', *, *, #5426, .T. ) ;
#4977=ORIENTED_EDGE ( 'NONE', *, *, #2105, .T. ) ;
#4983=EDGE_CURVE ( 'NONE', #6772, #2948, #2299, .T. ) ;
#4996=ADVANCED_FACE ( 'NONE', ( #2990 ), #8151, .F. ) ;
#5003=CARTESIAN_POINT ( 'NONE',  ( -105.0000000000000000, 105.0000000000000284, 240.0000000000000284 ) ) ;
#5004=ORIENTED_EDGE ( 'NONE', *, *, #6741, .F. ) ;
#5008=LINE ( 'NONE', #4361, #2160 ) ;
#5010=DIRECTION ( 'NONE',  ( -0.000000000000000000, 1.000000000000000000, -1.266875999117951024E-16 ) ) ;
#5013=EDGE_CURVE ( 'NONE', #7975, #3837, #5825, .T. ) ;
#5015=AXIS2_PLACEMENT_3D ( 'NONE', #6050, #7371, #265 ) ;
#5020=FACE_OUTER_BOUND ( 'NONE', #1951, .T. ) ;
#5024=VERTEX_POINT ( 'NONE', #5789 ) ;
#5027=DIRECTION ( 'NONE',  ( 1.000000000000000000, 0.000000000000000000, 0.000000000000000000 ) ) ;
#5037=AXIS2_PLACEMENT_3D ( 'NONE', #2898, #2782, #7942 ) ;
#5038=EDGE_CURVE ( 'NONE', #5777, #416, #3759, .T. ) ;
#5042=FACE_OUTER_BOUND ( 'NONE', #1671, .T. ) ;
#5056=PRODUCT ( 'Drive Unit', 'Drive Unit', '', ( #5531 ) ) ;
#5057=VERTEX_POINT ( 'NONE', #6404 ) ;
#5062=AXIS2_PLACEMENT_3D ( 'NONE', #4293, #7450, #6889 ) ;
#5063=EDGE_LOOP ( 'NONE', ( #267, #7039, #2411, #517 ) ) ;
#5079=AXIS2_PLACEMENT_3D ( 'NONE', #5458, #4013, #1539 ) ;
#5085=EDGE_CURVE ( 'NONE', #509, #3826, #2623, .T. ) ;
#5086=ORIENTED_EDGE ( 'NONE', *, *, #131, .F. ) ;
#5103=ORIENTED_EDGE ( 'NONE', *, *, #3549, .F. ) ;
#5116=AXIS2_PLACEMENT_3D ( 'NONE', #467, #422, #8063 ) ;
#5122=ORIENTED_EDGE ( 'NONE', *, *, #6299, .F. ) ;
#5125=DIRECTION ( 'NONE',  ( 0.000000000000000000, 0.000000000000000000, -1.000000000000000000 ) ) ;
#5137=ADVANCED_FACE ( 'NONE', ( #7744 ), #1961, .F. ) ;
#5140=VECTOR ( 'NONE', #6576, 1000.000000000000000 ) ;
#5146=DIRECTION ( 'NONE',  ( 1.000000000000000000, 0.000000000000000000, 0.000000000000000000 ) ) ;
#5150=CARTESIAN_POINT ( 'NONE',  ( -104.9999999999999432, -105.0000000000000853, 340.0000000000000000 ) ) ;
#5151=ADVANCED_FACE ( 'NONE', ( #3710 ), #8284, .F. ) ;
#5158=DIRECTION ( 'NONE',  ( -0.000000000000000000, -1.000000000000000000, -1.224646799147353207E-16 ) ) ;
#5168=EDGE_CURVE ( 'NONE', #5293, #5777, #5242, .T. ) ;
#5171=VECTOR ( 'NONE', #1571, 1000.000000000000000 ) ;
#5176=ORIENTED_EDGE ( 'NONE', *, *, #3022, .T. ) ;
#5179=VERTEX_POINT ( 'NONE', #109 ) ;
#5187=CARTESIAN_POINT ( 'NONE',  ( 0.000000000000000000, -125.0000000000000568, 66.99999999999997158 ) ) ;
#5190=DIRECTION ( 'NONE',  ( 2.643388153869419325E-16, -1.000000000000000000, -0.000000000000000000 ) ) ;
#5191=ORIENTED_EDGE ( 'NONE', *, *, #4577, .F. ) ;
#5192=ADVANCED_FACE ( 'NONE', ( #3923 ), #6623, .F. ) ;
#5216=ORIENTED_EDGE ( 'NONE', *, *, #7636, .F. ) ;
#5221=ORIENTED_EDGE ( 'NONE', *, *, #1357, .T. ) ;
#5230=CIRCLE ( 'NONE', #5633, 12.99999999999999822 ) ;
#5237=LINE ( 'NONE', #5280, #679 ) ;
#5242=CIRCLE ( 'NONE', #4824, 12.99999999999999822 ) ;
#5245=DIRECTION ( 'NONE',  ( -0.8571673007021116675, 1.049727191138617833E-16, 0.5150380749100552658 ) ) ;
#5252=DIRECTION ( 'NONE',  ( 1.000000000000000000, 0.000000000000000000, 0.000000000000000000 ) ) ;
#5256=ORIENTED_EDGE ( 'NONE', *, *, #6708, .T. ) ;
#5259=CARTESIAN_POINT ( 'NONE',  ( 55.00000000000000000, -55.00000000000000000, 240.0000000000000284 ) ) ;
#5268=DIRECTION ( 'NONE',  ( 1.000000000000000000, 0.000000000000000000, 0.000000000000000000 ) ) ;
#5271=VERTEX_POINT ( 'NONE', #5397 ) ;
#5273=FACE_OUTER_BOUND ( 'NONE', #1238, .T. ) ;
#5277=DIRECTION ( 'NONE',  ( 0.8571673007021116675, 0.000000000000000000, 0.5150380749100552658 ) ) ;
#5278=DIRECTION ( 'NONE',  ( 1.000000000000000000, 0.000000000000000000, 0.000000000000000000 ) ) ;
#5280=CARTESIAN_POINT ( 'NONE',  ( -50.00000000000000711, -55.00000000000000000, 220.0000000000000284 ) ) ;
#5282=CIRCLE ( 'NONE', #3797, 4.999999999999997335 ) ;
#5283=ORIENTED_EDGE ( 'NONE', *, *, #7636, .T. ) ;
#5284=FACE_OUTER_BOUND ( 'NONE', #2206, .T. ) ;
#5291=CARTESIAN_POINT ( 'NONE',  ( -105.0000000000000000, 72.49999999999997158, 19.99999999999998934 ) ) ;
#5292=DIRECTION ( 'NONE',  ( -0.000000000000000000, -0.000000000000000000, 1.000000000000000000 ) ) ;
#5293=VERTEX_POINT ( 'NONE', #4841 ) ;
#5301=CIRCLE ( 'NONE', #2858, 4.999999999999997335 ) ;
#5302=ORIENTED_EDGE ( 'NONE', *, *, #2868, .F. ) ;
#5305=EDGE_CURVE ( 'NONE', #1946, #1562, #8134, .T. ) ;
#5310=LINE ( 'NONE', #3952, #8346 ) ;
#5320=LINE ( 'NONE', #6021, #8323 ) ;
#5327=CARTESIAN_POINT ( 'NONE',  ( 0.000000000000000000, 52.49999999999997868, 66.99999999999994316 ) ) ;
#5333=DIRECTION ( 'NONE',  ( 1.000000000000000000, 0.000000000000000000, 0.000000000000000000 ) ) ;
#5335=DIRECTION ( 'NONE',  ( 1.000000000000000000, 0.000000000000000000, 0.000000000000000000 ) ) ;
#5341=ORIENTED_EDGE ( 'NONE', *, *, #3484, .F. ) ;
#5342=VECTOR ( 'NONE', #6553, 1000.000000000000000 ) ;
#5343=VERTEX_POINT ( 'NONE', #6231 ) ;
#5344=CARTESIAN_POINT ( 'NONE',  ( -125.0000000000000000, 125.0000000000000568, -9.184850993605156622E-15 ) ) ;
#5345=DIRECTION ( 'NONE',  ( 0.000000000000000000, 1.460819769243626884E-16, -1.000000000000000000 ) ) ;
#5347=LINE ( 'NONE', #2284, #3694 ) ;
#5349=EDGE_LOOP ( 'NONE', ( #4189, #7875, #5813, #2244 ) ) ;
#5354=EDGE_CURVE ( 'NONE', #5384, #6772, #359, .T. ) ;
#5357=DIRECTION ( 'NONE',  ( -0.000000000000000000, -0.000000000000000000, 1.000000000000000000 ) ) ;
#5361=CARTESIAN_POINT ( 'NONE',  ( 0.000000000000000000, -72.49999999999998579, 79.99999999999995737 ) ) ;
#5362=VECTOR ( 'NONE', #5391, 1000.000000000000000 ) ;
#5371=ORIENTED_EDGE ( 'NONE', *, *, #7000, .T. ) ;
#5375=VECTOR ( 'NONE', #7374, 1000.000000000000000 ) ;
#5377=DIRECTION ( 'NONE',  ( -0.000000000000000000, -1.000000000000000000, -1.224646799147353207E-16 ) ) ;
#5384=VERTEX_POINT ( 'NONE', #3515 ) ;
#5391=DIRECTION ( 'NONE',  ( -0.000000000000000000, -1.000000000000000000, 1.586032892321652236E-16 ) ) ;
#5395=VERTEX_POINT ( 'NONE', #4114 ) ;
#5396=VERTEX_POINT ( 'NONE', #1050 ) ;
#5397=CARTESIAN_POINT ( 'NONE',  ( 110.0000000000000142, 115.0000000000000000, 340.0000000000000000 ) ) ;
#5398=EDGE_LOOP ( 'NONE', ( #5779, #358, #4464, #1637 ) ) ;
#5401=LINE ( 'NONE', #2857, #7712 ) ;
#5421=FACE_OUTER_BOUND ( 'NONE', #3023, .T. ) ;
#5426=EDGE_CURVE ( 'NONE', #323, #549, #1723, .T. ) ;
#5431=LINE ( 'NONE', #3783, #7272 ) ;
#5434=CARTESIAN_POINT ( 'NONE',  ( -125.0000000000000000, -52.50000000000000000, 190.0000000000000284 ) ) ;
#5443=VERTEX_POINT ( 'NONE', #3188 ) ;
#5446=AXIS2_PLACEMENT_3D ( 'NONE', #2004, #7194, #1416 ) ;
#5451=EDGE_CURVE ( 'NONE', #1904, #3406, #5008, .T. ) ;
#5454=ORIENTED_EDGE ( 'NONE', *, *, #461, .T. ) ;
#5457=ORIENTED_EDGE ( 'NONE', *, *, #443, .T. ) ;
#5458=CARTESIAN_POINT ( 'NONE',  ( 115.0000000000000000, 115.0000000000000000, 340.0000000000000000 ) ) ;
#5460=EDGE_LOOP ( 'NONE', ( #6846, #4135 ) ) ;
#5484=DIRECTION ( 'NONE',  ( 1.000000000000000000, 1.321694076934710648E-16, 0.000000000000000000 ) ) ;
#5486=CIRCLE ( 'NONE', #6419, 12.99999999999999822 ) ;
#5509=DIRECTION ( 'NONE',  ( -0.000000000000000000, -1.000000000000000000, 1.586032892321652236E-16 ) ) ;
#5516=LINE ( 'NONE', #6771, #6724 ) ;
#5518=FACE_OUTER_BOUND ( 'NONE', #2326, .T. ) ;
#5521=EDGE_LOOP ( 'NONE', ( #3009, #5283, #2970, #2419 ) ) ;
#5523=VECTOR ( 'NONE', #6895, 1000.000000000000000 ) ;
#5526=EDGE_LOOP ( 'NONE', ( #651, #4062, #6993, #4140 ) ) ;
#5530=PLANE ( 'NONE',  #2936 ) ;
#5531=PRODUCT_CONTEXT ( 'NONE', #6285, 'mechanical' ) ;
#5537=EDGE_CURVE ( 'NONE', #1211, #5443, #2534, .T. ) ;
#5539=VERTEX_POINT ( 'NONE', #1950 ) ;
#5542=ORIENTED_EDGE ( 'NONE', *, *, #6013, .F. ) ;
#5545=DIRECTION ( 'NONE',  ( 0.000000000000000000, 0.000000000000000000, 1.000000000000000000 ) ) ;
#5546=DIRECTION ( 'NONE',  ( 0.000000000000000000, 0.000000000000000000, 1.000000000000000000 ) ) ;
#5547=ORIENTED_EDGE ( 'NONE', *, *, #385, .F. ) ;
#5557=CARTESIAN_POINT ( 'NONE',  ( 115.0000000000000000, 115.0000000000000000, 270.0000000000000000 ) ) ;
#5564=CARTESIAN_POINT ( 'NONE',  ( 125.0000000000000000, -52.50000000000000000, 190.0000000000000284 ) ) ;
#5565=CIRCLE ( 'NONE', #7872, 4.999999999999990230 ) ;
#5582=LINE ( 'NONE', #3872, #923 ) ;
#5596=CARTESIAN_POINT ( 'NONE',  ( 0.000000000000000000, -52.49999999999996447, 66.99999999999995737 ) ) ;
#5612=DIRECTION ( 'NONE',  ( 1.000000000000000000, -0.000000000000000000, 0.000000000000000000 ) ) ;
#5630=LINE ( 'NONE', #1796, #5523 ) ;
#5633=AXIS2_PLACEMENT_3D ( 'NONE', #690, #5158, #1247 ) ;
#5641=CARTESIAN_POINT ( 'NONE',  ( 125.0000000000000000, 125.0000000000000568, 19.99999999999998934 ) ) ;
#5645=CARTESIAN_POINT ( 'NONE',  ( 125.0000000000000000, -125.0000000000000000, 340.0000000000000000 ) ) ;
#5646=VERTEX_POINT ( 'NONE', #7926 ) ;
#5652=FACE_OUTER_BOUND ( 'NONE', #8080, .T. ) ;
#5656=CARTESIAN_POINT ( 'NONE',  ( 125.0000000000000000, 125.0000000000000568, -9.184850993605156622E-15 ) ) ;
#5661=AXIS2_PLACEMENT_3D ( 'NONE', #2784, #4005, #896 ) ;
#5665=CIRCLE ( 'NONE', #4573, 12.99999999999999822 ) ;
#5667=STYLED_ITEM('',(#8386),#6502);
#5670=VERTEX_POINT ( 'NONE', #6570 ) ;
#5671=EDGE_CURVE ( 'NONE', #314, #2572, #7125, .T. ) ;
#5676=CARTESIAN_POINT ( 'NONE',  ( -105.0000000000000000, 105.0000000000000284, 340.0000000000000000 ) ) ;
#5677=ORIENTED_EDGE ( 'NONE', *, *, #510, .F. ) ;
#5681=DIRECTION ( 'NONE',  ( 1.000000000000000000, 0.000000000000000000, 0.000000000000000000 ) ) ;
#5688=EDGE_CURVE ( 'NONE', #952, #469, #100, .T. ) ;
#5710=DIRECTION ( 'NONE',  ( -0.000000000000000000, -0.000000000000000000, 1.000000000000000000 ) ) ;
#5711=AXIS2_PLACEMENT_3D ( 'NONE', #5641, #1289, #3176 ) ;
#5714=ORIENTED_EDGE ( 'NONE', *, *, #1804, .F. ) ;
#5715=PLANE ( 'NONE',  #2653 ) ;
#5720=AXIS2_PLACEMENT_3D ( 'NONE', #7294, #221, #2245 ) ;
#5725=AXIS2_PLACEMENT_3D ( 'NONE', #5968, #3500, #5335 ) ;
#5728=EDGE_LOOP ( 'NONE', ( #1353, #1862 ) ) ;
#5734=ORIENTED_EDGE ( 'NONE', *, *, #7394, .F. ) ;
#5736=EDGE_CURVE ( 'NONE', #5293, #6212, #3421, .T. ) ;
#5739=EDGE_LOOP ( 'NONE', ( #2057, #6943, #5542, #3606 ) ) ;
#5742=CARTESIAN_POINT ( 'NONE',  ( 125.0000000000000000, 125.0000000000000000, 340.0000000000000000 ) ) ;
#5746=CIRCLE ( 'NONE', #2124, 4.999999999999990230 ) ;
#5760=ORIENTED_EDGE ( 'NONE', *, *, #5354, .T. ) ;
#5765=CARTESIAN_POINT ( 'NONE',  ( -110.0000000000000142, 115.0000000000000000, 340.0000000000000000 ) ) ;
#5772=VECTOR ( 'NONE', #4414, 1000.000000000000000 ) ;
#5774=ADVANCED_FACE ( 'NONE', ( #4181 ), #8039, .F. ) ;
#5775=VERTEX_POINT ( 'NONE', #3504 ) ;
#5776=AXIS2_PLACEMENT_3D ( 'NONE', #1429, #2158, #145 ) ;
#5777=VERTEX_POINT ( 'NONE', #2843 ) ;
#5779=ORIENTED_EDGE ( 'NONE', *, *, #3154, .T. ) ;
#5783=EDGE_LOOP ( 'NONE', ( #8065, #7347, #8049, #8012 ) ) ;
#5789=CARTESIAN_POINT ( 'NONE',  ( 1.592040838891560279E-15, 72.49999999999995737, 92.99999999999994316 ) ) ;
#5790=ORIENTED_EDGE ( 'NONE', *, *, #7751, .T. ) ;
#5791=DIRECTION ( 'NONE',  ( 1.000000000000000000, 0.000000000000000000, 0.000000000000000000 ) ) ;
#5792=CIRCLE ( 'NONE', #7687, 4.999999999999990230 ) ;
#5793=CARTESIAN_POINT ( 'NONE',  ( 50.00000000000000000, 55.00000000000000000, 240.0000000000000284 ) ) ;
#5796=EDGE_CURVE ( 'NONE', #6702, #7449, #266, .T. ) ;
#5797=CARTESIAN_POINT ( 'NONE',  ( 0.000000000000000000, -72.49999999999997158, 20.00000000000001776 ) ) ;
#5799=MECHANICAL_DESIGN_GEOMETRIC_PRESENTATION_REPRESENTATION('',(#5667),#541);
#5802=LINE ( 'NONE', #6300, #2131 ) ;
#5807=DIRECTION ( 'NONE',  ( 1.000000000000000000, 0.000000000000000000, 0.000000000000000000 ) ) ;
#5808=DIRECTION ( 'NONE',  ( 0.000000000000000000, -1.000000000000000000, 1.586032892321652236E-16 ) ) ;
#5813=ORIENTED_EDGE ( 'NONE', *, *, #2105, .F. ) ;
#5816=ORIENTED_EDGE ( 'NONE', *, *, #5671, .F. ) ;
#5819=CARTESIAN_POINT ( 'NONE',  ( -105.0000000000000000, 105.0000000000000284, 340.0000000000000000 ) ) ;
#5821=EDGE_CURVE ( 'NONE', #5539, #5396, #5516, .T. ) ;
#5823=PLANE ( 'NONE',  #4454 ) ;
#5825=LINE ( 'NONE', #5742, #5772 ) ;
#5828=EDGE_CURVE ( 'NONE', #7656, #4494, #6861, .T. ) ;
#5832=LINE ( 'NONE', #5793, #6962 ) ;
#5845=DIRECTION ( 'NONE',  ( 1.000000000000000000, 0.000000000000000000, 0.000000000000000000 ) ) ;
#5846=DIRECTION ( 'NONE',  ( 1.000000000000000000, 0.000000000000000000, 0.000000000000000000 ) ) ;
#5857=DIRECTION ( 'NONE',  ( 0.000000000000000000, 0.000000000000000000, -1.000000000000000000 ) ) ;
#5858=AXIS2_PLACEMENT_3D ( 'NONE', #344, #262, #6045 ) ;
#5867=CARTESIAN_POINT ( 'NONE',  ( -115.0000000000000000, -115.0000000000000000, 340.0000000000000000 ) ) ;
#5870=EDGE_CURVE ( 'NONE', #624, #5179, #525, .T. ) ;
#5873=DIRECTION ( 'NONE',  ( 0.000000000000000000, 0.000000000000000000, 1.000000000000000000 ) ) ;
#5877=FACE_OUTER_BOUND ( 'NONE', #7681, .T. ) ;
#5884=CARTESIAN_POINT ( 'NONE',  ( 0.000000000000000000, 0.000000000000000000, 0.000000000000000000 ) ) ;
#5887=ORIENTED_EDGE ( 'NONE', *, *, #4563, .T. ) ;
#5896=DIRECTION ( 'NONE',  ( -0.000000000000000000, -0.000000000000000000, 1.000000000000000000 ) ) ;
#5898=DIRECTION ( 'NONE',  ( 1.000000000000000000, 0.000000000000000000, 0.000000000000000000 ) ) ;
#5906=AXIS2_PLACEMENT_3D ( 'NONE', #3987, #62, #3268 ) ;
#5909=VERTEX_POINT ( 'NONE', #4867 ) ;
#5910=LINE ( 'NONE', #1489, #7672 ) ;
#5920=ADVANCED_FACE ( 'NONE', ( #1551 ), #4603, .F. ) ;
#5921=ORIENTED_EDGE ( 'NONE', *, *, #5038, .T. ) ;
#5923=VECTOR ( 'NONE', #162, 1000.000000000000000 ) ;
#5924=DIRECTION ( 'NONE',  ( -0.000000000000000000, -0.000000000000000000, 1.000000000000000000 ) ) ;
#5927=DIRECTION ( 'NONE',  ( 1.000000000000000000, 0.000000000000000000, 0.000000000000000000 ) ) ;
#5936=ORIENTED_EDGE ( 'NONE', *, *, #3135, .F. ) ;
#5938=CARTESIAN_POINT ( 'NONE',  ( 1.592040838891559490E-15, 125.0000000000000568, 92.99999999999992895 ) ) ;
#5940=EDGE_CURVE ( 'NONE', #6702, #5539, #1893, .T. ) ;
#5949=CARTESIAN_POINT ( 'NONE',  ( -55.00000000000000711, -55.00000000000000000, 216.9956969048622284 ) ) ;
#5950=ORIENTED_EDGE ( 'NONE', *, *, #5796, .F. ) ;
#5956=DIRECTION ( 'NONE',  ( 0.000000000000000000, -1.000000000000000000, -1.224646799147353207E-16 ) ) ;
#5959=DIRECTION ( 'NONE',  ( 1.000000000000000000, 0.000000000000000000, 0.000000000000000000 ) ) ;
#5961=VECTOR ( 'NONE', #6839, 1000.000000000000000 ) ;
#5963=DIRECTION ( 'NONE',  ( -1.000000000000000000, -0.000000000000000000, -0.000000000000000000 ) ) ;
#5968=CARTESIAN_POINT ( 'NONE',  ( -55.00000000000000000, 55.00000000000000000, 220.0000000000000284 ) ) ;
#5970=FACE_BOUND ( 'NONE', #5460, .T. ) ;
#5972=EDGE_CURVE ( 'NONE', #5396, #7449, #3092, .T. ) ;
#5983=CARTESIAN_POINT ( 'NONE',  ( 0.000000000000000000, -105.0000000000000711, 79.99999999999997158 ) ) ;
#5986=LINE ( 'NONE', #2775, #7550 ) ;
#5989=CARTESIAN_POINT ( 'NONE',  ( -105.0000000000000000, 72.50000000000000000, -212.5000000000000568 ) ) ;
#6000=CARTESIAN_POINT ( 'NONE',  ( 0.000000000000000000, -72.49999999999998579, 79.99999999999995737 ) ) ;
#6011=EDGE_CURVE ( 'NONE', #3478, #4879, #691, .T. ) ;
#6013=EDGE_CURVE ( 'NONE', #6134, #3849, #7688, .T. ) ;
#6021=CARTESIAN_POINT ( 'NONE',  ( 110.0000000000000142, 115.0000000000000000, 340.0000000000000000 ) ) ;
#6023=CARTESIAN_POINT ( 'NONE',  ( 120.0000000000000000, 115.0000000000000000, 270.0000000000000000 ) ) ;
#6029=FACE_BOUND ( 'NONE', #6333, .T. ) ;
#6030=DIRECTION ( 'NONE',  ( 1.000000000000000000, 0.000000000000000000, 0.000000000000000000 ) ) ;
#6031=PLANE ( 'NONE',  #2175 ) ;
#6034=AXIS2_PLACEMENT_3D ( 'NONE', #1312, #8325, #3879 ) ;
#6037=ORIENTED_EDGE ( 'NONE', *, *, #2088, .T. ) ;
#6045=DIRECTION ( 'NONE',  ( 1.000000000000000000, 0.000000000000000000, 0.000000000000000000 ) ) ;
#6047=CIRCLE ( 'NONE', #5661, 4.999999999999990230 ) ;
#6050=CARTESIAN_POINT ( 'NONE',  ( 0.000000000000000000, -52.49999999999996447, 79.99999999999995737 ) ) ;
#6055=DIRECTION ( 'NONE',  ( 1.000000000000000000, -0.000000000000000000, 0.000000000000000000 ) ) ;
#6057=FACE_OUTER_BOUND ( 'NONE', #6680, .T. ) ;
#6071=LINE ( 'NONE', #287, #3395 ) ;
#6074=EDGE_CURVE ( 'NONE', #3690, #5057, #6047, .T. ) ;
#6075=ORIENTED_EDGE ( 'NONE', *, *, #1806, .F. ) ;
#6080=ORIENTED_EDGE ( 'NONE', *, *, #2322, .T. ) ;
#6081=CARTESIAN_POINT ( 'NONE',  ( 0.000000000000000000, 72.49999999999994316, 240.0000000000000284 ) ) ;
#6083=DIRECTION ( 'NONE',  ( -0.000000000000000000, -0.000000000000000000, 1.000000000000000000 ) ) ;
#6098=CARTESIAN_POINT ( 'NONE',  ( 125.0000000000000000, -125.0000000000000000, 340.0000000000000000 ) ) ;
#6100=FACE_OUTER_BOUND ( 'NONE', #3130, .T. ) ;
#6123=EDGE_CURVE ( 'NONE', #8125, #1093, #3491, .T. ) ;
#6134=VERTEX_POINT ( 'NONE', #5327 ) ;
#6138=EDGE_CURVE ( 'NONE', #5179, #624, #6730, .T. ) ;
#6141=EDGE_LOOP ( 'NONE', ( #2760, #7312, #7605, #3038 ) ) ;
#6143=EDGE_LOOP ( 'NONE', ( #3719, #1722 ) ) ;
#6144=FACE_BOUND ( 'NONE', #6599, .T. ) ;
#6148=CIRCLE ( 'NONE', #8329, 4.999999999999990230 ) ;
#6150=CARTESIAN_POINT ( 'NONE',  ( 125.0000000000000000, 52.50000000000000000, 190.0000000000000284 ) ) ;
#6156=ORIENTED_EDGE ( 'NONE', *, *, #6011, .F. ) ;
#6168=EDGE_LOOP ( 'NONE', ( #2305, #3650, #711, #4559 ) ) ;
#6171=AXIS2_PLACEMENT_3D ( 'NONE', #5361, #4724, #817 ) ;
#6178=DIRECTION ( 'NONE',  ( 1.000000000000000000, 0.000000000000000000, 0.000000000000000000 ) ) ;
#6184=CONICAL_SURFACE ( 'NONE', #2432, 4.999999999999990230, 1.029744258676653201 ) ;
#6187=ORIENTED_EDGE ( 'NONE', *, *, #6894, .F. ) ;
#6188=AXIS2_PLACEMENT_3D ( 'NONE', #2113, #2642, #4571 ) ;
#6192=ORIENTED_EDGE ( 'NONE', *, *, #3549, .T. ) ;
#6197=AXIS2_PLACEMENT_3D ( 'NONE', #1324, #3971, #3933 ) ;
#6211=CARTESIAN_POINT ( 'NONE',  ( -50.00000000000000711, 55.00000000000000000, 220.0000000000000284 ) ) ;
#6212=VERTEX_POINT ( 'NONE', #373 ) ;
#6214=AXIS2_PLACEMENT_3D ( 'NONE', #4713, #4150, #3427 ) ;
#6222=DIRECTION ( 'NONE',  ( 0.000000000000000000, 0.000000000000000000, -1.000000000000000000 ) ) ;
#6224=ORIENTED_EDGE ( 'NONE', *, *, #3122, .F. ) ;
#6226=DIRECTION ( 'NONE',  ( -0.000000000000000000, -0.000000000000000000, 1.000000000000000000 ) ) ;
#6231=CARTESIAN_POINT ( 'NONE',  ( -50.00000000000000000, 55.00000000000000000, 240.0000000000000284 ) ) ;
#6235=CYLINDRICAL_SURFACE ( 'NONE', #4272, 12.99999999999999822 ) ;
#6237=VERTEX_POINT ( 'NONE', #1110 ) ;
#6242=CARTESIAN_POINT ( 'NONE',  ( -110.0000000000000142, 115.0000000000000000, 270.0000000000000000 ) ) ;
#6247=ORIENTED_EDGE ( 'NONE', *, *, #3572, .T. ) ;
#6248=ORIENTED_EDGE ( 'NONE', *, *, #2026, .F. ) ;
#6249=VERTEX_POINT ( 'NONE', #3529 ) ;
#6258=ORIENTED_EDGE ( 'NONE', *, *, #2032, .T. ) ;
#6266=FACE_BOUND ( 'NONE', #5728, .T. ) ;
#6271=CARTESIAN_POINT ( 'NONE',  ( 105.0000000000000000, 105.0000000000000711, 340.0000000000000000 ) ) ;
#6272=ORIENTED_EDGE ( 'NONE', *, *, #6975, .F. ) ;
#6276=VERTEX_POINT ( 'NONE', #3568 ) ;
#6285=APPLICATION_CONTEXT ( 'automotive_design' ) ;
#6295=CARTESIAN_POINT ( 'NONE',  ( 0.000000000000000000, 125.0000000000000568, 79.99999999999992895 ) ) ;
#6299=EDGE_CURVE ( 'NONE', #3768, #5024, #255, .T. ) ;
#6300=CARTESIAN_POINT ( 'NONE',  ( -120.0000000000000000, -115.0000000000000000, 340.0000000000000000 ) ) ;
#6303=VECTOR ( 'NONE', #1279, 1000.000000000000000 ) ;
#6319=ORIENTED_EDGE ( 'NONE', *, *, #2323, .T. ) ;
#6320=UNCERTAINTY_MEASURE_WITH_UNIT (LENGTH_MEASURE( 1.000000000000000082E-05 ), #4638, 'distance_accuracy_value', 'NONE');
#6324=AXIS2_PLACEMENT_3D ( 'NONE', #348, #2921, #6178 ) ;
#6327=CARTESIAN_POINT ( 'NONE',  ( 105.0000000000000000, 72.49999999999997158, 19.99999999999998934 ) ) ;
#6331=CIRCLE ( 'NONE', #2691, 4.999999999999997335 ) ;
#6333=EDGE_LOOP ( 'NONE', ( #1325, #4496 ) ) ;
#6335=CARTESIAN_POINT ( 'NONE',  ( 115.0000000000000000, 115.0000000000000000, 340.0000000000000000 ) ) ;
#6337=DIRECTION ( 'NONE',  ( -0.000000000000000000, -0.000000000000000000, 1.000000000000000000 ) ) ;
#6349=FACE_OUTER_BOUND ( 'NONE', #7715, .T. ) ;
#6350=ADVANCED_FACE ( 'NONE', ( #2543 ), #7420, .F. ) ;
#6355=CARTESIAN_POINT ( 'NONE',  ( -125.0000000000000000, -125.0000000000000568, -9.184850993605156622E-15 ) ) ;
#6361=CARTESIAN_POINT ( 'NONE',  ( 125.0000000000000000, 125.0000000000000568, -9.184850993605156622E-15 ) ) ;
#6364=CARTESIAN_POINT ( 'NONE',  ( 125.0000000000000000, 125.0000000000000568, 19.99999999999998934 ) ) ;
#6371=EDGE_CURVE ( 'NONE', #7416, #7579, #2625, .T. ) ;
#6373=EDGE_CURVE ( 'NONE', #8146, #5670, #1875, .T. ) ;
#6378=EDGE_CURVE ( 'NONE', #5057, #3690, #120, .T. ) ;
#6380=EDGE_LOOP ( 'NONE', ( #5936, #909 ) ) ;
#6389=DIRECTION ( 'NONE',  ( 1.000000000000000000, 0.000000000000000000, 0.000000000000000000 ) ) ;
#6400=ADVANCED_FACE ( 'NONE', ( #7014, #5020 ), #6406, .F. ) ;
#6402=CARTESIAN_POINT ( 'NONE',  ( 120.0000000000000000, -115.0000000000000000, 270.0000000000000000 ) ) ;
#6403=CARTESIAN_POINT ( 'NONE',  ( -120.0000000000000000, -115.0000000000000000, 270.0000000000000000 ) ) ;
#6404=CARTESIAN_POINT ( 'NONE',  ( -110.0000000000000142, -115.0000000000000000, 340.0000000000000000 ) ) ;
#6406=PLANE ( 'NONE',  #1082 ) ;
#6408=ORIENTED_EDGE ( 'NONE', *, *, #2088, .F. ) ;
#6410=ORIENTED_EDGE ( 'NONE', *, *, #5671, .T. ) ;
#6412=DIRECTION ( 'NONE',  ( -0.8571673007021116675, 1.049727191138617833E-16, 0.5150380749100552658 ) ) ;
#6419=AXIS2_PLACEMENT_3D ( 'NONE', #1775, #4317, #1122 ) ;
#6424=VECTOR ( 'NONE', #7575, 1000.000000000000000 ) ;
#6427=CARTESIAN_POINT ( 'NONE',  ( 115.0000000000000000, 115.0000000000000000, 340.0000000000000000 ) ) ;
#6463=DIRECTION ( 'NONE',  ( 1.000000000000000000, 0.000000000000000000, 0.000000000000000000 ) ) ;
#6465=DIRECTION ( 'NONE',  ( 1.000000000000000000, 0.000000000000000000, 0.000000000000000000 ) ) ;
#6468=ORIENTED_EDGE ( 'NONE', *, *, #3585, .F. ) ;
#6471=DIRECTION ( 'NONE',  ( -0.000000000000000000, -0.000000000000000000, 1.000000000000000000 ) ) ;
#6478=DIRECTION ( 'NONE',  ( -0.000000000000000000, -0.000000000000000000, 1.000000000000000000 ) ) ;
#6479=ORIENTED_EDGE ( 'NONE', *, *, #2430, .T. ) ;
#6490=EDGE_CURVE ( 'NONE', #1935, #5539, #5237, .T. ) ;
#6495=DIRECTION ( 'NONE',  ( 0.000000000000000000, 1.000000000000000000, -1.632680918566406547E-16 ) ) ;
#6496=ORIENTED_EDGE ( 'NONE', *, *, #3122, .T. ) ;
#6501=ORIENTED_EDGE ( 'NONE', *, *, #7540, .F. ) ;
#6502=MANIFOLD_SOLID_BREP ( 'Cut-Extrude4', #2230 ) ;
#6504=PLANE ( 'NONE',  #3749 ) ;
#6517=AXIS2_PLACEMENT_3D ( 'NONE', #2177, #7308, #852 ) ;
#6526=CARTESIAN_POINT ( 'NONE',  ( 125.0000000000000000, -125.0000000000000568, -9.184850993605156622E-15 ) ) ;
#6529=CARTESIAN_POINT ( 'NONE',  ( 105.0000000000000000, -72.49999999999994316, -212.5000000000000568 ) ) ;
#6532=DIRECTION ( 'NONE',  ( 0.000000000000000000, 0.000000000000000000, 1.000000000000000000 ) ) ;
#6533=ORIENTED_EDGE ( 'NONE', *, *, #7797, .F. ) ;
#6552=ORIENTED_EDGE ( 'NONE', *, *, #4983, .F. ) ;
#6553=DIRECTION ( 'NONE',  ( 2.643388153869419325E-16, -1.000000000000000000, -0.000000000000000000 ) ) ;
#6570=CARTESIAN_POINT ( 'NONE',  ( -104.9999999999999432, -105.0000000000000853, 340.0000000000000000 ) ) ;
#6571=AXIS2_PLACEMENT_3D ( 'NONE', #7922, #3542, #4704 ) ;
#6574=DIRECTION ( 'NONE',  ( 1.000000000000000000, 0.000000000000000000, 0.000000000000000000 ) ) ;
#6575=AXIS2_PLACEMENT_3D ( 'NONE', #3240, #7048, #5146 ) ;
#6576=DIRECTION ( 'NONE',  ( -1.000000000000000000, -0.000000000000000000, -0.000000000000000000 ) ) ;
#6579=VECTOR ( 'NONE', #6969, 1000.000000000000000 ) ;
#6580=VERTEX_POINT ( 'NONE', #8015 ) ;
#6583=ORIENTED_EDGE ( 'NONE', *, *, #3482, .F. ) ;
#6593=DIRECTION ( 'NONE',  ( -0.000000000000000000, -1.000000000000000000, -0.000000000000000000 ) ) ;
#6594=PLANE ( 'NONE',  #3680 ) ;
#6598=DIRECTION ( 'NONE',  ( -0.000000000000000000, -0.000000000000000000, 1.000000000000000000 ) ) ;
#6599=EDGE_LOOP ( 'NONE', ( #2339, #3775 ) ) ;
#6602=ADVANCED_FACE ( 'NONE', ( #6100 ), #6235, .F. ) ;
#6605=DIRECTION ( 'NONE',  ( 1.000000000000000000, 0.000000000000000000, 0.000000000000000000 ) ) ;
#6610=CIRCLE ( 'NONE', #6197, 12.99999999999999822 ) ;
#6613=VERTEX_POINT ( 'NONE', #4193 ) ;
#6619=DIRECTION ( 'NONE',  ( -0.000000000000000000, -0.000000000000000000, 1.000000000000000000 ) ) ;
#6623=CYLINDRICAL_SURFACE ( 'NONE', #8212, 4.999999999999990230 ) ;
#6624=ORIENTED_EDGE ( 'NONE', *, *, #5736, .T. ) ;
#6628=LINE ( 'NONE', #3397, #7202 ) ;
#6633=DIRECTION ( 'NONE',  ( -0.000000000000000000, -0.000000000000000000, 1.000000000000000000 ) ) ;
#6634=ADVANCED_FACE ( 'NONE', ( #4320, #6144 ), #5530, .F. ) ;
#6641=FACE_OUTER_BOUND ( 'NONE', #3180, .T. ) ;
#6645=DIRECTION ( 'NONE',  ( -0.000000000000000000, -0.000000000000000000, 1.000000000000000000 ) ) ;
#6655=ORIENTED_EDGE ( 'NONE', *, *, #7807, .F. ) ;
#6657=LINE ( 'NONE', #224, #8217 ) ;
#6658=LINE ( 'NONE', #225, #2416 ) ;
#6660=VECTOR ( 'NONE', #7981, 1000.000000000000000 ) ;
#6661=ORIENTED_EDGE ( 'NONE', *, *, #4642, .F. ) ;
#6664=ORIENTED_EDGE ( 'NONE', *, *, #5013, .T. ) ;
#6672=CARTESIAN_POINT ( 'NONE',  ( 125.0000000000000000, -125.0000000000000568, -9.184850993605156622E-15 ) ) ;
#6676=FACE_BOUND ( 'NONE', #7992, .T. ) ;
#6679=EDGE_LOOP ( 'NONE', ( #1816, #5302, #4088, #841 ) ) ;
#6680=EDGE_LOOP ( 'NONE', ( #7376, #7165, #193 ) ) ;
#6690=DIRECTION ( 'NONE',  ( 1.000000000000000000, 0.000000000000000000, 0.000000000000000000 ) ) ;
#6693=CARTESIAN_POINT ( 'NONE',  ( 0.000000000000000000, 72.49999999999997158, 19.99999999999998934 ) ) ;
#6702=VERTEX_POINT ( 'NONE', #2458 ) ;
#6704=CIRCLE ( 'NONE', #1591, 4.999999999999990230 ) ;
#6705=CIRCLE ( 'NONE', #6571, 4.999999999999997335 ) ;
#6708=EDGE_CURVE ( 'NONE', #1008, #7975, #3114, .T. ) ;
#6717=VECTOR ( 'NONE', #4710, 1000.000000000000000 ) ;
#6722=DIRECTION ( 'NONE',  ( -1.321694076934710155E-16, 1.000000000000000000, 0.000000000000000000 ) ) ;
#6724=VECTOR ( 'NONE', #2280, 1000.000000000000000 ) ;
#6730=CIRCLE ( 'NONE', #7274, 4.999999999999990230 ) ;
#6732=VERTEX_POINT ( 'NONE', #4490 ) ;
#6737=VECTOR ( 'NONE', #5190, 1000.000000000000000 ) ;
#6739=DIRECTION ( 'NONE',  ( -0.000000000000000000, 1.000000000000000000, -0.000000000000000000 ) ) ;
#6741=EDGE_CURVE ( 'NONE', #2457, #5775, #4554, .T. ) ;
#6748=ORIENTED_EDGE ( 'NONE', *, *, #4437, .F. ) ;
#6757=CARTESIAN_POINT ( 'NONE',  ( 54.99999999999999289, 55.00000000000000000, 216.9956969048622284 ) ) ;
#6759=ORIENTED_EDGE ( 'NONE', *, *, #7362, .F. ) ;
#6769=VECTOR ( 'NONE', #8131, 1000.000000000000000 ) ;
#6770=EDGE_LOOP ( 'NONE', ( #2864, #2006 ) ) ;
#6771=CARTESIAN_POINT ( 'NONE',  ( -50.00000000000000000, -55.00000000000000000, 240.0000000000000284 ) ) ;
#6772=VERTEX_POINT ( 'NONE', #2496 ) ;
#6774=CARTESIAN_POINT ( 'NONE',  ( 50.00000000000000000, 55.00000000000000000, 240.0000000000000284 ) ) ;
#6780=ORIENTED_EDGE ( 'NONE', *, *, #7157, .F. ) ;
#6800=CARTESIAN_POINT ( 'NONE',  ( -105.0000000000000000, -105.0000000000000568, 20.00000000000004619 ) ) ;
#6803=ORIENTED_EDGE ( 'NONE', *, *, #5821, .T. ) ;
#6821=AXIS2_PLACEMENT_3D ( 'NONE', #2717, #1459, #214 ) ;
#6822=DIRECTION ( 'NONE',  ( -0.000000000000000000, -0.000000000000000000, 1.000000000000000000 ) ) ;
#6833=ORIENTED_EDGE ( 'NONE', *, *, #5013, .F. ) ;
#6835=CARTESIAN_POINT ( 'NONE',  ( -104.9999999999999432, -105.0000000000000853, 340.0000000000000000 ) ) ;
#6837=DIRECTION ( 'NONE',  ( 1.000000000000000000, 0.000000000000000000, 0.000000000000000000 ) ) ;
#6839=DIRECTION ( 'NONE',  ( -0.8571673007021134438, 1.049727191138620051E-16, 0.5150380749100522682 ) ) ;
#6846=ORIENTED_EDGE ( 'NONE', *, *, #2860, .T. ) ;
#6848=CARTESIAN_POINT ( 'NONE',  ( -125.0000000000000000, -125.0000000000000568, -9.184850993605156622E-15 ) ) ;
#6853=EDGE_CURVE ( 'NONE', #6276, #6237, #1350, .T. ) ;
#6861=LINE ( 'NONE', #2880, #7133 ) ;
#6864=DIRECTION ( 'NONE',  ( -0.000000000000000000, -0.000000000000000000, 1.000000000000000000 ) ) ;
#6870=AXIS2_PLACEMENT_3D ( 'NONE', #5867, #4416, #1964 ) ;
#6871=ORIENTED_EDGE ( 'NONE', *, *, #4577, .T. ) ;
#6883=ORIENTED_EDGE ( 'NONE', *, *, #5821, .F. ) ;
#6889=DIRECTION ( 'NONE',  ( 1.000000000000000000, 0.000000000000000000, 0.000000000000000000 ) ) ;
#6891=AXIS2_PLACEMENT_3D ( 'NONE', #3437, #4163, #2334 ) ;
#6892=CARTESIAN_POINT ( 'NONE',  ( 105.0000000000000000, -72.49999999999994316, 20.00000000000002842 ) ) ;
#6894=EDGE_CURVE ( 'NONE', #1112, #5179, #5310, .T. ) ;
#6895=DIRECTION ( 'NONE',  ( 0.000000000000000000, 1.000000000000000000, 0.000000000000000000 ) ) ;
#6898=CIRCLE ( 'NONE', #4731, 4.999999999999990230 ) ;
#6905=ADVANCED_FACE ( 'NONE', ( #7296 ), #1428, .F. ) ;
#6919=CARTESIAN_POINT ( 'NONE',  ( -115.0000000000000000, 115.0000000000000000, 270.0000000000000000 ) ) ;
#6935=EDGE_LOOP ( 'NONE', ( #5103, #5004, #6037, #7446 ) ) ;
#6943=ORIENTED_EDGE ( 'NONE', *, *, #3079, .T. ) ;
#6950=CARTESIAN_POINT ( 'NONE',  ( -60.00000000000000000, 55.00000000000000000, 240.0000000000000284 ) ) ;
#6953=VERTEX_POINT ( 'NONE', #5344 ) ;
#6956=DIRECTION ( 'NONE',  ( -0.000000000000000000, -0.000000000000000000, 1.000000000000000000 ) ) ;
#6962=VECTOR ( 'NONE', #8290, 1000.000000000000000 ) ;
#6968=ORIENTED_EDGE ( 'NONE', *, *, #3430, .F. ) ;
#6969=DIRECTION ( 'NONE',  ( -0.000000000000000000, -0.000000000000000000, 1.000000000000000000 ) ) ;
#6975=EDGE_CURVE ( 'NONE', #5646, #2109, #7891, .T. ) ;
#6978=DIRECTION ( 'NONE',  ( 1.000000000000000000, 0.000000000000000000, 0.000000000000000000 ) ) ;
#6979=AXIS2_PLACEMENT_3D ( 'NONE', #6000, #345, #4096 ) ;
#6981=EDGE_LOOP ( 'NONE', ( #7146, #2167, #7772 ) ) ;
#6993=ORIENTED_EDGE ( 'NONE', *, *, #1283, .F. ) ;
#6996=ORIENTED_EDGE ( 'NONE', *, *, #1643, .F. ) ;
#7000=EDGE_CURVE ( 'NONE', #8106, #5384, #6657, .T. ) ;
#7013=ADVANCED_FACE ( 'NONE', ( #7856 ), #6184, .F. ) ;
#7014=FACE_BOUND ( 'NONE', #2492, .T. ) ;
#7021=CARTESIAN_POINT ( 'NONE',  ( 0.000000000000000000, 105.0000000000000426, 79.99999999999992895 ) ) ;
#7023=ADVANCED_FACE ( 'NONE', ( #4627 ), #3507, .F. ) ;
#7024=CARTESIAN_POINT ( 'NONE',  ( 115.0000000000000000, -115.0000000000000000, 340.0000000000000000 ) ) ;
#7026=DIRECTION ( 'NONE',  ( -0.000000000000000000, -0.000000000000000000, 1.000000000000000000 ) ) ;
#7028=DIRECTION ( 'NONE',  ( 1.000000000000000000, 0.000000000000000000, 0.000000000000000000 ) ) ;
#7030=VECTOR ( 'NONE', #8092, 1000.000000000000000 ) ;
#7036=CYLINDRICAL_SURFACE ( 'NONE', #2407, 4.999999999999997335 ) ;
#7039=ORIENTED_EDGE ( 'NONE', *, *, #4164, .T. ) ;
#7048=DIRECTION ( 'NONE',  ( -0.000000000000000000, -0.000000000000000000, 1.000000000000000000 ) ) ;
#7051=EDGE_CURVE ( 'NONE', #717, #4180, #2882, .T. ) ;
#7061=FACE_OUTER_BOUND ( 'NONE', #3227, .T. ) ;
#7068=AXIS2_PLACEMENT_3D ( 'NONE', #3902, #6471, #5845 ) ;
#7083=DIRECTION ( 'NONE',  ( -0.000000000000000000, -0.000000000000000000, 1.000000000000000000 ) ) ;
#7087=CONICAL_SURFACE ( 'NONE', #5062, 4.999999999999990230, 1.029744258676653201 ) ;
#7096=CIRCLE ( 'NONE', #2031, 4.999999999999990230 ) ;
#7102=DIRECTION ( 'NONE',  ( -0.000000000000000000, -1.460819769243626884E-16, -1.000000000000000000 ) ) ;
#7103=ADVANCED_FACE ( 'NONE', ( #3464 ), #4972, .F. ) ;
#7105=DIRECTION ( 'NONE',  ( 0.000000000000000000, 0.000000000000000000, -1.000000000000000000 ) ) ;
#7106=EDGE_CURVE ( 'NONE', #4879, #1112, #5792, .T. ) ;
#7111=LINE ( 'NONE', #3939, #907 ) ;
#7113=FACE_OUTER_BOUND ( 'NONE', #2468, .T. ) ;
#7115=ADVANCED_FACE ( 'NONE', ( #5518 ), #1672, .F. ) ;
#7122=EDGE_LOOP ( 'NONE', ( #1630, #7902, #368, #1355 ) ) ;
#7125=LINE ( 'NONE', #6526, #7679 ) ;
#7131=CARTESIAN_POINT ( 'NONE',  ( 55.00000000000000000, -55.00000000000000000, 220.0000000000000284 ) ) ;
#7133=VECTOR ( 'NONE', #4747, 1000.000000000000000 ) ;
#7137=EDGE_CURVE ( 'NONE', #8125, #1878, #8176, .T. ) ;
#7143=AXIS2_PLACEMENT_3D ( 'NONE', #3129, #3043, #1249 ) ;
#7146=ORIENTED_EDGE ( 'NONE', *, *, #6490, .F. ) ;
#7147=LINE ( 'NONE', #2787, #5342 ) ;
#7152=CARTESIAN_POINT ( 'NONE',  ( 125.0000000000000000, 125.0000000000000000, 340.0000000000000000 ) ) ;
#7155=FACE_OUTER_BOUND ( 'NONE', #2319, .T. ) ;
#7157=EDGE_CURVE ( 'NONE', #2948, #8106, #4955, .T. ) ;
#7161=EDGE_CURVE ( 'NONE', #314, #952, #5431, .T. ) ;
#7165=ORIENTED_EDGE ( 'NONE', *, *, #152, .T. ) ;
#7166=DIRECTION ( 'NONE',  ( -1.000000000000000000, -0.000000000000000000, -0.000000000000000000 ) ) ;
#7181=CARTESIAN_POINT ( 'NONE',  ( 50.00000000000000711, -55.00000000000000000, 220.0000000000000284 ) ) ;
#7186=CARTESIAN_POINT ( 'NONE',  ( 55.00000000000000000, 55.00000000000000000, 220.0000000000000284 ) ) ;
#7188=DIRECTION ( 'NONE',  ( -0.000000000000000000, -0.000000000000000000, 1.000000000000000000 ) ) ;
#7193=FACE_OUTER_BOUND ( 'NONE', #7325, .T. ) ;
#7194=DIRECTION ( 'NONE',  ( -0.000000000000000000, -0.000000000000000000, 1.000000000000000000 ) ) ;
#7196=CYLINDRICAL_SURFACE ( 'NONE', #4421, 4.999999999999990230 ) ;
#7202=VECTOR ( 'NONE', #199, 1000.000000000000000 ) ;
#7203=SHAPE_REPRESENTATION ( 'Drive Unit', ( #1299 ), #205 ) ;
#7211=ADVANCED_FACE ( 'NONE', ( #5042 ), #657, .T. ) ;
#7216=EDGE_CURVE ( 'NONE', #416, #6212, #1213, .T. ) ;
#7219=CARTESIAN_POINT ( 'NONE',  ( -125.0000000000000000, -52.49999999999997158, 0.000000000000000000 ) ) ;
#7221=CYLINDRICAL_SURFACE ( 'NONE', #1597, 4.999999999999997335 ) ;
#7222=FACE_OUTER_BOUND ( 'NONE', #4315, .T. ) ;
#7227=ORIENTED_EDGE ( 'NONE', *, *, #3331, .T. ) ;
#7228=LINE ( 'NONE', #168, #7367 ) ;
#7232=CONICAL_SURFACE ( 'NONE', #2393, 4.999999999999990230, 1.029744258676653201 ) ;
#7248=CIRCLE ( 'NONE', #7666, 4.999999999999990230 ) ;
#7257=DIRECTION ( 'NONE',  ( -0.000000000000000000, -0.000000000000000000, 1.000000000000000000 ) ) ;
#7264=VECTOR ( 'NONE', #2536, 1000.000000000000000 ) ;
#7272=VECTOR ( 'NONE', #4479, 1000.000000000000000 ) ;
#7274=AXIS2_PLACEMENT_3D ( 'NONE', #7909, #2708, #6030 ) ;
#7292=ADVANCED_FACE ( 'NONE', ( #7155 ), #7196, .F. ) ;
#7294=CARTESIAN_POINT ( 'NONE',  ( -55.00000000000000000, 55.00000000000000000, 220.0000000000000284 ) ) ;
#7295=ORIENTED_EDGE ( 'NONE', *, *, #5940, .F. ) ;
#7296=FACE_OUTER_BOUND ( 'NONE', #3589, .T. ) ;
#7300=VECTOR ( 'NONE', #2539, 1000.000000000000000 ) ;
#7306=DIRECTION ( 'NONE',  ( -0.000000000000000000, -1.000000000000000000, 1.586032892321652236E-16 ) ) ;
#7308=DIRECTION ( 'NONE',  ( -0.000000000000000000, -0.000000000000000000, 1.000000000000000000 ) ) ;
#7312=ORIENTED_EDGE ( 'NONE', *, *, #461, .F. ) ;
#7315=EDGE_LOOP ( 'NONE', ( #4962, #5122, #1297, #2758 ) ) ;
#7316=AXIS2_PLACEMENT_3D ( 'NONE', #6295, #1840, #2176 ) ;
#7321=DIRECTION ( 'NONE',  ( 1.000000000000000000, 0.000000000000000000, 0.000000000000000000 ) ) ;
#7322=( NAMED_UNIT ( * ) SI_UNIT ( $, .STERADIAN. ) SOLID_ANGLE_UNIT ( ) );
#7325=EDGE_LOOP ( 'NONE', ( #5547, #963, #6247 ) ) ;
#7332=ORIENTED_EDGE ( 'NONE', *, *, #4536, .T. ) ;
#7333=DIRECTION ( 'NONE',  ( 1.000000000000000000, 0.000000000000000000, 0.000000000000000000 ) ) ;
#7343=DIRECTION ( 'NONE',  ( 0.000000000000000000, 1.000000000000000000, 0.000000000000000000 ) ) ;
#7345=( NAMED_UNIT ( * ) SI_UNIT ( $, .STERADIAN. ) SOLID_ANGLE_UNIT ( ) );
#7347=ORIENTED_EDGE ( 'NONE', *, *, #1343, .F. ) ;
#7350=CARTESIAN_POINT ( 'NONE',  ( 120.0000000000000000, 115.0000000000000000, 340.0000000000000000 ) ) ;
#7356=FACE_OUTER_BOUND ( 'NONE', #7592, .T. ) ;
#7357=ORIENTED_EDGE ( 'NONE', *, *, #8312, .T. ) ;
#7359=LINE ( 'NONE', #6403, #5961 ) ;
#7362=EDGE_CURVE ( 'NONE', #8240, #1008, #3338, .T. ) ;
#7367=VECTOR ( 'NONE', #2020, 1000.000000000000000 ) ;
#7371=DIRECTION ( 'NONE',  ( 0.000000000000000000, -1.000000000000000000, -1.460819769243626884E-16 ) ) ;
#7372=EDGE_CURVE ( 'NONE', #952, #1918, #4017, .T. ) ;
#7374=DIRECTION ( 'NONE',  ( -0.000000000000000000, -0.000000000000000000, 1.000000000000000000 ) ) ;
#7376=ORIENTED_EDGE ( 'NONE', *, *, #2164, .F. ) ;
#7383=VECTOR ( 'NONE', #6412, 1000.000000000000000 ) ;
#7389=AXIS2_PLACEMENT_3D ( 'NONE', #7021, #730, #7619 ) ;
#7391=CONICAL_SURFACE ( 'NONE', #1877, 4.999999999999990230, 1.029744258676653201 ) ;
#7394=EDGE_CURVE ( 'NONE', #7579, #5443, #6331, .T. ) ;
#7407=AXIS2_PLACEMENT_3D ( 'NONE', #4910, #4870, #1042 ) ;
#7416=VERTEX_POINT ( 'NONE', #3412 ) ;
#7420=CONICAL_SURFACE ( 'NONE', #1622, 4.999999999999990230, 1.029744258676656754 ) ;
#7433=ORIENTED_EDGE ( 'NONE', *, *, #7216, .F. ) ;
#7438=ADVANCED_FACE ( 'NONE', ( #7113 ), #4612, .F. ) ;
#7442=CIRCLE ( 'NONE', #9, 4.999999999999997335 ) ;
#7443=ORIENTED_EDGE ( 'NONE', *, *, #4836, .F. ) ;
#7446=ORIENTED_EDGE ( 'NONE', *, *, #6378, .T. ) ;
#7449=VERTEX_POINT ( 'NONE', #701 ) ;
#7450=DIRECTION ( 'NONE',  ( -0.000000000000000000, -0.000000000000000000, 1.000000000000000000 ) ) ;
#7467=ORIENTED_EDGE ( 'NONE', *, *, #1759, .T. ) ;
#7478=LINE ( 'NONE', #6023, #3914 ) ;
#7480=ADVANCED_FACE ( 'NONE', ( #8076 ), #3536, .F. ) ;
#7487=VERTEX_POINT ( 'NONE', #2795 ) ;
#7490=EDGE_LOOP ( 'NONE', ( #1648, #7498 ) ) ;
#7497=DIRECTION ( 'NONE',  ( -0.000000000000000000, -0.000000000000000000, 1.000000000000000000 ) ) ;
#7498=ORIENTED_EDGE ( 'NONE', *, *, #6138, .F. ) ;
#7503=ORIENTED_EDGE ( 'NONE', *, *, #1647, .T. ) ;
#7504=CIRCLE ( 'NONE', #3047, 12.99999999999999822 ) ;
#7510=ORIENTED_EDGE ( 'NONE', *, *, #3641, .T. ) ;
#7512=VECTOR ( 'NONE', #436, 1000.000000000000000 ) ;
#7529=EDGE_CURVE ( 'NONE', #1904, #6580, #2349, .T. ) ;
#7535=ORIENTED_EDGE ( 'NONE', *, *, #3189, .T. ) ;
#7540=EDGE_CURVE ( 'NONE', #5777, #5293, #5665, .T. ) ;
#7550=VECTOR ( 'NONE', #5357, 1000.000000000000000 ) ;
#7551=FACE_BOUND ( 'NONE', #6770, .T. ) ;
#7562=AXIS2_PLACEMENT_3D ( 'NONE', #2106, #6598, #821 ) ;
#7572=CARTESIAN_POINT ( 'NONE',  ( -55.00000000000000711, 55.00000000000000000, 216.9956969048622284 ) ) ;
#7575=DIRECTION ( 'NONE',  ( -0.000000000000000000, -1.632680918566406547E-16, -1.000000000000000000 ) ) ;
#7577=DIRECTION ( 'NONE',  ( -0.000000000000000000, -1.000000000000000000, 1.586032892321652236E-16 ) ) ;
#7579=VERTEX_POINT ( 'NONE', #4772 ) ;
#7592=EDGE_LOOP ( 'NONE', ( #3793, #884, #3241, #7963 ) ) ;
#7596=EDGE_LOOP ( 'NONE', ( #6655, #82, #6080, #4903 ) ) ;
#7605=ORIENTED_EDGE ( 'NONE', *, *, #5537, .T. ) ;
#7609=ORIENTED_EDGE ( 'NONE', *, *, #1486, .T. ) ;
#7616=VECTOR ( 'NONE', #5277, 1000.000000000000000 ) ;
#7619=DIRECTION ( 'NONE',  ( 0.000000000000000000, 0.000000000000000000, -1.000000000000000000 ) ) ;
#7630=CARTESIAN_POINT ( 'NONE',  ( 0.000000000000000000, -125.0000000000000568, 79.99999999999997158 ) ) ;
#7636=EDGE_CURVE ( 'NONE', #3982, #4695, #5630, .T. ) ;
#7637=ORIENTED_EDGE ( 'NONE', *, *, #5354, .F. ) ;
#7656=VERTEX_POINT ( 'NONE', #4385 ) ;
#7663=AXIS2_PLACEMENT_3D ( 'NONE', #4736, #3450, #954 ) ;
#7666=AXIS2_PLACEMENT_3D ( 'NONE', #2251, #6822, #1676 ) ;
#7667=CARTESIAN_POINT ( 'NONE',  ( 125.0000000000000000, -52.50000000000000000, 190.0000000000000284 ) ) ;
#7668=PLANE ( 'NONE',  #7143 ) ;
#7670=FACE_BOUND ( 'NONE', #3048, .T. ) ;
#7672=VECTOR ( 'NONE', #815, 1000.000000000000000 ) ;
#7677=DIRECTION ( 'NONE',  ( 0.000000000000000000, 0.000000000000000000, -1.000000000000000000 ) ) ;
#7679=VECTOR ( 'NONE', #7166, 1000.000000000000000 ) ;
#7681=EDGE_LOOP ( 'NONE', ( #2281, #3753, #7357, #1520 ) ) ;
#7682=CARTESIAN_POINT ( 'NONE',  ( -55.00000000000000000, 55.00000000000000000, 220.0000000000000284 ) ) ;
#7687=AXIS2_PLACEMENT_3D ( 'NONE', #1716, #439, #8004 ) ;
#7688=CIRCLE ( 'NONE', #1475, 12.99999999999999822 ) ;
#7689=ORIENTED_EDGE ( 'NONE', *, *, #6123, .F. ) ;
#7700=EDGE_LOOP ( 'NONE', ( #4937, #1737, #7227, #7503 ) ) ;
#7702=AXIS2_PLACEMENT_3D ( 'NONE', #7186, #5292, #774 ) ;
#7703=ADVANCED_FACE ( 'NONE', ( #477 ), #8165, .F. ) ;
#7704=EDGE_CURVE ( 'NONE', #4085, #5395, #1753, .T. ) ;
#7708=CARTESIAN_POINT ( 'NONE',  ( 125.0000000000000000, 52.49999999999997158, 0.000000000000000000 ) ) ;
#7712=VECTOR ( 'NONE', #977, 1000.000000000000000 ) ;
#7715=EDGE_LOOP ( 'NONE', ( #1342, #3770, #524 ) ) ;
#7718=ADVANCED_FACE ( 'NONE', ( #7061, #3847 ), #7668, .T. ) ;
#7734=ORIENTED_EDGE ( 'NONE', *, *, #5828, .F. ) ;
#7739=LINE ( 'NONE', #6402, #7300 ) ;
#7741=VECTOR ( 'NONE', #6593, 1000.000000000000000 ) ;
#7744=FACE_OUTER_BOUND ( 'NONE', #6168, .T. ) ;
#7747=DIRECTION ( 'NONE',  ( 0.000000000000000000, 1.632680918566406547E-16, 1.000000000000000000 ) ) ;
#7751=EDGE_CURVE ( 'NONE', #549, #8146, #3724, .T. ) ;
#7756=CARTESIAN_POINT ( 'NONE',  ( 125.0000000000000000, 52.49999999999997158, 0.000000000000000000 ) ) ;
#7758=CIRCLE ( 'NONE', #5446, 4.999999999999990230 ) ;
#7769=ORIENTED_EDGE ( 'NONE', *, *, #6371, .T. ) ;
#7772=ORIENTED_EDGE ( 'NONE', *, *, #5940, .T. ) ;
#7774=EDGE_LOOP ( 'NONE', ( #3562, #6624, #580, #427 ) ) ;
#7797=EDGE_CURVE ( 'NONE', #4180, #7487, #1451, .T. ) ;
#7799=EDGE_LOOP ( 'NONE', ( #1228, #5677, #7535, #6075 ) ) ;
#7805=DIRECTION ( 'NONE',  ( -0.000000000000000000, -0.000000000000000000, 1.000000000000000000 ) ) ;
#7807=EDGE_CURVE ( 'NONE', #448, #5909, #816, .T. ) ;
#7813=AXIS2_PLACEMENT_3D ( 'NONE', #4587, #3714, #5857 ) ;
#7817=DIRECTION ( 'NONE',  ( 0.000000000000000000, 1.000000000000000000, -1.266875999117951024E-16 ) ) ;
#7829=DIRECTION ( 'NONE',  ( 0.8571673007021116675, 0.000000000000000000, 0.5150380749100552658 ) ) ;
#7830=VECTOR ( 'NONE', #7102, 1000.000000000000000 ) ;
#7856=FACE_OUTER_BOUND ( 'NONE', #6981, .T. ) ;
#7859=CARTESIAN_POINT ( 'NONE',  ( -110.0000000000000142, -115.0000000000000000, 270.0000000000000000 ) ) ;
#7861=LINE ( 'NONE', #1960, #7616 ) ;
#7864=DIRECTION ( 'NONE',  ( 0.8571673007021116675, 0.000000000000000000, 0.5150380749100552658 ) ) ;
#7872=AXIS2_PLACEMENT_3D ( 'NONE', #1690, #4802, #6837 ) ;
#7874=CYLINDRICAL_SURFACE ( 'NONE', #7562, 4.999999999999997335 ) ;
#7875=ORIENTED_EDGE ( 'NONE', *, *, #6975, .T. ) ;
#7881=DIRECTION ( 'NONE',  ( 1.000000000000000000, 0.000000000000000000, 0.000000000000000000 ) ) ;
#7883=CONICAL_SURFACE ( 'NONE', #6517, 4.999999999999990230, 1.029744258676656754 ) ;
#7885=CARTESIAN_POINT ( 'NONE',  ( 0.000000000000000000, 125.0000000000000568, 79.99999999999992895 ) ) ;
#7891=LINE ( 'NONE', #5938, #6717 ) ;
#7892=DIRECTION ( 'NONE',  ( 1.000000000000000000, 0.000000000000000000, 0.000000000000000000 ) ) ;
#7895=CARTESIAN_POINT ( 'NONE',  ( -125.0000000000000000, 0.000000000000000000, 0.000000000000000000 ) ) ;
#7897=EDGE_CURVE ( 'NONE', #5646, #4085, #6610, .T. ) ;
#7902=ORIENTED_EDGE ( 'NONE', *, *, #3920, .F. ) ;
#7909=CARTESIAN_POINT ( 'NONE',  ( -115.0000000000000000, 115.0000000000000000, 340.0000000000000000 ) ) ;
#7920=VECTOR ( 'NONE', #762, 1000.000000000000000 ) ;
#7921=CARTESIAN_POINT ( 'NONE',  ( -115.0000000000000000, -115.0000000000000000, 340.0000000000000000 ) ) ;
#7922=CARTESIAN_POINT ( 'NONE',  ( -55.00000000000000000, -55.00000000000000000, 240.0000000000000284 ) ) ;
#7926=CARTESIAN_POINT ( 'NONE',  ( 1.592040838891560279E-15, 125.0000000000000568, 92.99999999999992895 ) ) ;
#7929=DIRECTION ( 'NONE',  ( 0.000000000000000000, -1.224646799147353207E-16, 1.000000000000000000 ) ) ;
#7931=FACE_OUTER_BOUND ( 'NONE', #2081, .T. ) ;
#7932=AXIS2_PLACEMENT_3D ( 'NONE', #879, #6619, #6574 ) ;
#7938=ADVANCED_FACE ( 'NONE', ( #123 ), #7874, .F. ) ;
#7942=DIRECTION ( 'NONE',  ( 0.000000000000000000, 0.000000000000000000, -1.000000000000000000 ) ) ;
#7951=CYLINDRICAL_SURFACE ( 'NONE', #1709, 4.999999999999990230 ) ;
#7963=ORIENTED_EDGE ( 'NONE', *, *, #2268, .T. ) ;
#7969=CARTESIAN_POINT ( 'NONE',  ( 125.0000000000000000, -52.50000000000000000, 190.0000000000000284 ) ) ;
#7975=VERTEX_POINT ( 'NONE', #5656 ) ;
#7981=DIRECTION ( 'NONE',  ( -0.000000000000000000, 1.000000000000000000, -1.266875999117951024E-16 ) ) ;
#7992=EDGE_LOOP ( 'NONE', ( #4113, #3610 ) ) ;
#7994=PRODUCT_DEFINITION_FORMATION_WITH_SPECIFIED_SOURCE ( 'ANY', '', #5056, .NOT_KNOWN. ) ;
#7997=DIRECTION ( 'NONE',  ( 1.000000000000000000, 0.000000000000000000, 0.000000000000000000 ) ) ;
#7998=VECTOR ( 'NONE', #876, 1000.000000000000000 ) ;
#8004=DIRECTION ( 'NONE',  ( 1.000000000000000000, 0.000000000000000000, 0.000000000000000000 ) ) ;
#8007=CARTESIAN_POINT ( 'NONE',  ( 115.0000000000000000, -115.0000000000000000, 270.0000000000000000 ) ) ;
#8010=ORIENTED_EDGE ( 'NONE', *, *, #1921, .T. ) ;
#8012=ORIENTED_EDGE ( 'NONE', *, *, #7372, .T. ) ;
#8015=CARTESIAN_POINT ( 'NONE',  ( -50.00000000000000711, 55.00000000000000000, 220.0000000000000284 ) ) ;
#8023=DIRECTION ( 'NONE',  ( 0.000000000000000000, -1.266875999117951024E-16, 1.000000000000000000 ) ) ;
#8030=ADVANCED_FACE ( 'NONE', ( #7356 ), #6031, .F. ) ;
#8039=CYLINDRICAL_SURFACE ( 'NONE', #2297, 4.999999999999990230 ) ;
#8046=DIRECTION ( 'NONE',  ( -0.000000000000000000, -0.000000000000000000, 1.000000000000000000 ) ) ;
#8049=ORIENTED_EDGE ( 'NONE', *, *, #5688, .F. ) ;
#8053=EDGE_CURVE ( 'NONE', #4879, #624, #2982, .T. ) ;
#8063=DIRECTION ( 'NONE',  ( 0.000000000000000000, 0.000000000000000000, 1.000000000000000000 ) ) ;
#8065=ORIENTED_EDGE ( 'NONE', *, *, #4825, .T. ) ;
#8068=ORIENTED_EDGE ( 'NONE', *, *, #7137, .T. ) ;
#8071=ORIENTED_EDGE ( 'NONE', *, *, #7704, .T. ) ;
#8073=AXIS2_PLACEMENT_3D ( 'NONE', #5557, #2359, #1001 ) ;
#8076=FACE_OUTER_BOUND ( 'NONE', #4110, .T. ) ;
#8080=EDGE_LOOP ( 'NONE', ( #6156, #7510, #1837 ) ) ;
#8089=LINE ( 'NONE', #2972, #74 ) ;
#8092=DIRECTION ( 'NONE',  ( -0.000000000000000000, -1.632680918566406547E-16, 1.000000000000000000 ) ) ;
#8094=ORIENTED_EDGE ( 'NONE', *, *, #6490, .T. ) ;
#8100=ORIENTED_EDGE ( 'NONE', *, *, #7106, .T. ) ;
#8106=VERTEX_POINT ( 'NONE', #6327 ) ;
#8108=CONICAL_SURFACE ( 'NONE', #1244, 4.999999999999990230, 1.029744258676653201 ) ;
#8125=VERTEX_POINT ( 'NONE', #630 ) ;
#8127=DIRECTION ( 'NONE',  ( -0.000000000000000000, -0.000000000000000000, 1.000000000000000000 ) ) ;
#8131=DIRECTION ( 'NONE',  ( -1.000000000000000000, -0.000000000000000000, -0.000000000000000000 ) ) ;
#8134=LINE ( 'NONE', #6098, #367 ) ;
#8140=EDGE_CURVE ( 'NONE', #1878, #5670, #3874, .T. ) ;
#8143=SHAPE_DEFINITION_REPRESENTATION ( #3786, #7203 ) ;
#8146=VERTEX_POINT ( 'NONE', #5819 ) ;
#8151=CYLINDRICAL_SURFACE ( 'NONE', #6575, 4.999999999999997335 ) ;
#8165=CYLINDRICAL_SURFACE ( 'NONE', #2438, 4.999999999999990230 ) ;
#8172=CARTESIAN_POINT ( 'NONE',  ( -125.0000000000000000, -125.0000000000000000, 340.0000000000000000 ) ) ;
#8174=CARTESIAN_POINT ( 'NONE',  ( -110.0000000000000142, 115.0000000000000000, 270.0000000000000000 ) ) ;
#8176=LINE ( 'NONE', #915, #944 ) ;
#8212=AXIS2_PLACEMENT_3D ( 'NONE', #804, #7257, #5278 ) ;
#8217=VECTOR ( 'NONE', #7817, 1000.000000000000000 ) ;
#8219=EDGE_CURVE ( 'NONE', #3826, #1534, #4659, .T. ) ;
#8221=DIRECTION ( 'NONE',  ( -0.000000000000000000, -0.000000000000000000, 1.000000000000000000 ) ) ;
#8240=VERTEX_POINT ( 'NONE', #2565 ) ;
#8243=EDGE_LOOP ( 'NONE', ( #5790, #2448, #7637, #3554 ) ) ;
#8246=LINE ( 'NONE', #1953, #4683 ) ;
#8253=DIRECTION ( 'NONE',  ( -1.000000000000000000, -1.321694076934710155E-16, -0.000000000000000000 ) ) ;
#8255=DIRECTION ( 'NONE',  ( -0.000000000000000000, -0.000000000000000000, 1.000000000000000000 ) ) ;
#8262=CARTESIAN_POINT ( 'NONE',  ( 0.000000000000000000, 125.0000000000000568, 66.99999999999992895 ) ) ;
#8269=ADVANCED_FACE ( 'NONE', ( #576 ), #1337, .F. ) ;
#8270=DIRECTION ( 'NONE',  ( 0.000000000000000000, 0.000000000000000000, -1.000000000000000000 ) ) ;
#8274=VERTEX_POINT ( 'NONE', #2035 ) ;
#8276=VERTEX_POINT ( 'NONE', #6950 ) ;
#8284=CYLINDRICAL_SURFACE ( 'NONE', #6034, 12.99999999999999822 ) ;
#8290=DIRECTION ( 'NONE',  ( -0.000000000000000000, -0.000000000000000000, 1.000000000000000000 ) ) ;
#8295=ORIENTED_EDGE ( 'NONE', *, *, #6138, .T. ) ;
#8310=ORIENTED_EDGE ( 'NONE', *, *, #6299, .T. ) ;
#8312=EDGE_CURVE ( 'NONE', #5271, #1665, #5746, .T. ) ;
#8323=VECTOR ( 'NONE', #4597, 1000.000000000000000 ) ;
#8325=DIRECTION ( 'NONE',  ( -0.000000000000000000, -1.000000000000000000, 1.586032892321652236E-16 ) ) ;
#8329=AXIS2_PLACEMENT_3D ( 'NONE', #699, #4477, #7028 ) ;
#8346=VECTOR ( 'NONE', #2655, 1000.000000000000000 ) ;
#8380=COLOUR_RGB('Light Blue',0.38,0.62,0.78);
#8381=FILL_AREA_STYLE_COLOUR('',#8380);
#8382=FILL_AREA_STYLE('',(#8381));
#8383=SURFACE_STYLE_FILL_AREA(#8382);
#8384=SURFACE_SIDE_STYLE('',(#8383));
#8385=SURFACE_STYLE_USAGE(.BOTH.,#8384);
#8386=PRESENTATION_STYLE_ASSIGNMENT((#8385));
ENDSEC;
END-ISO-10303-21;
